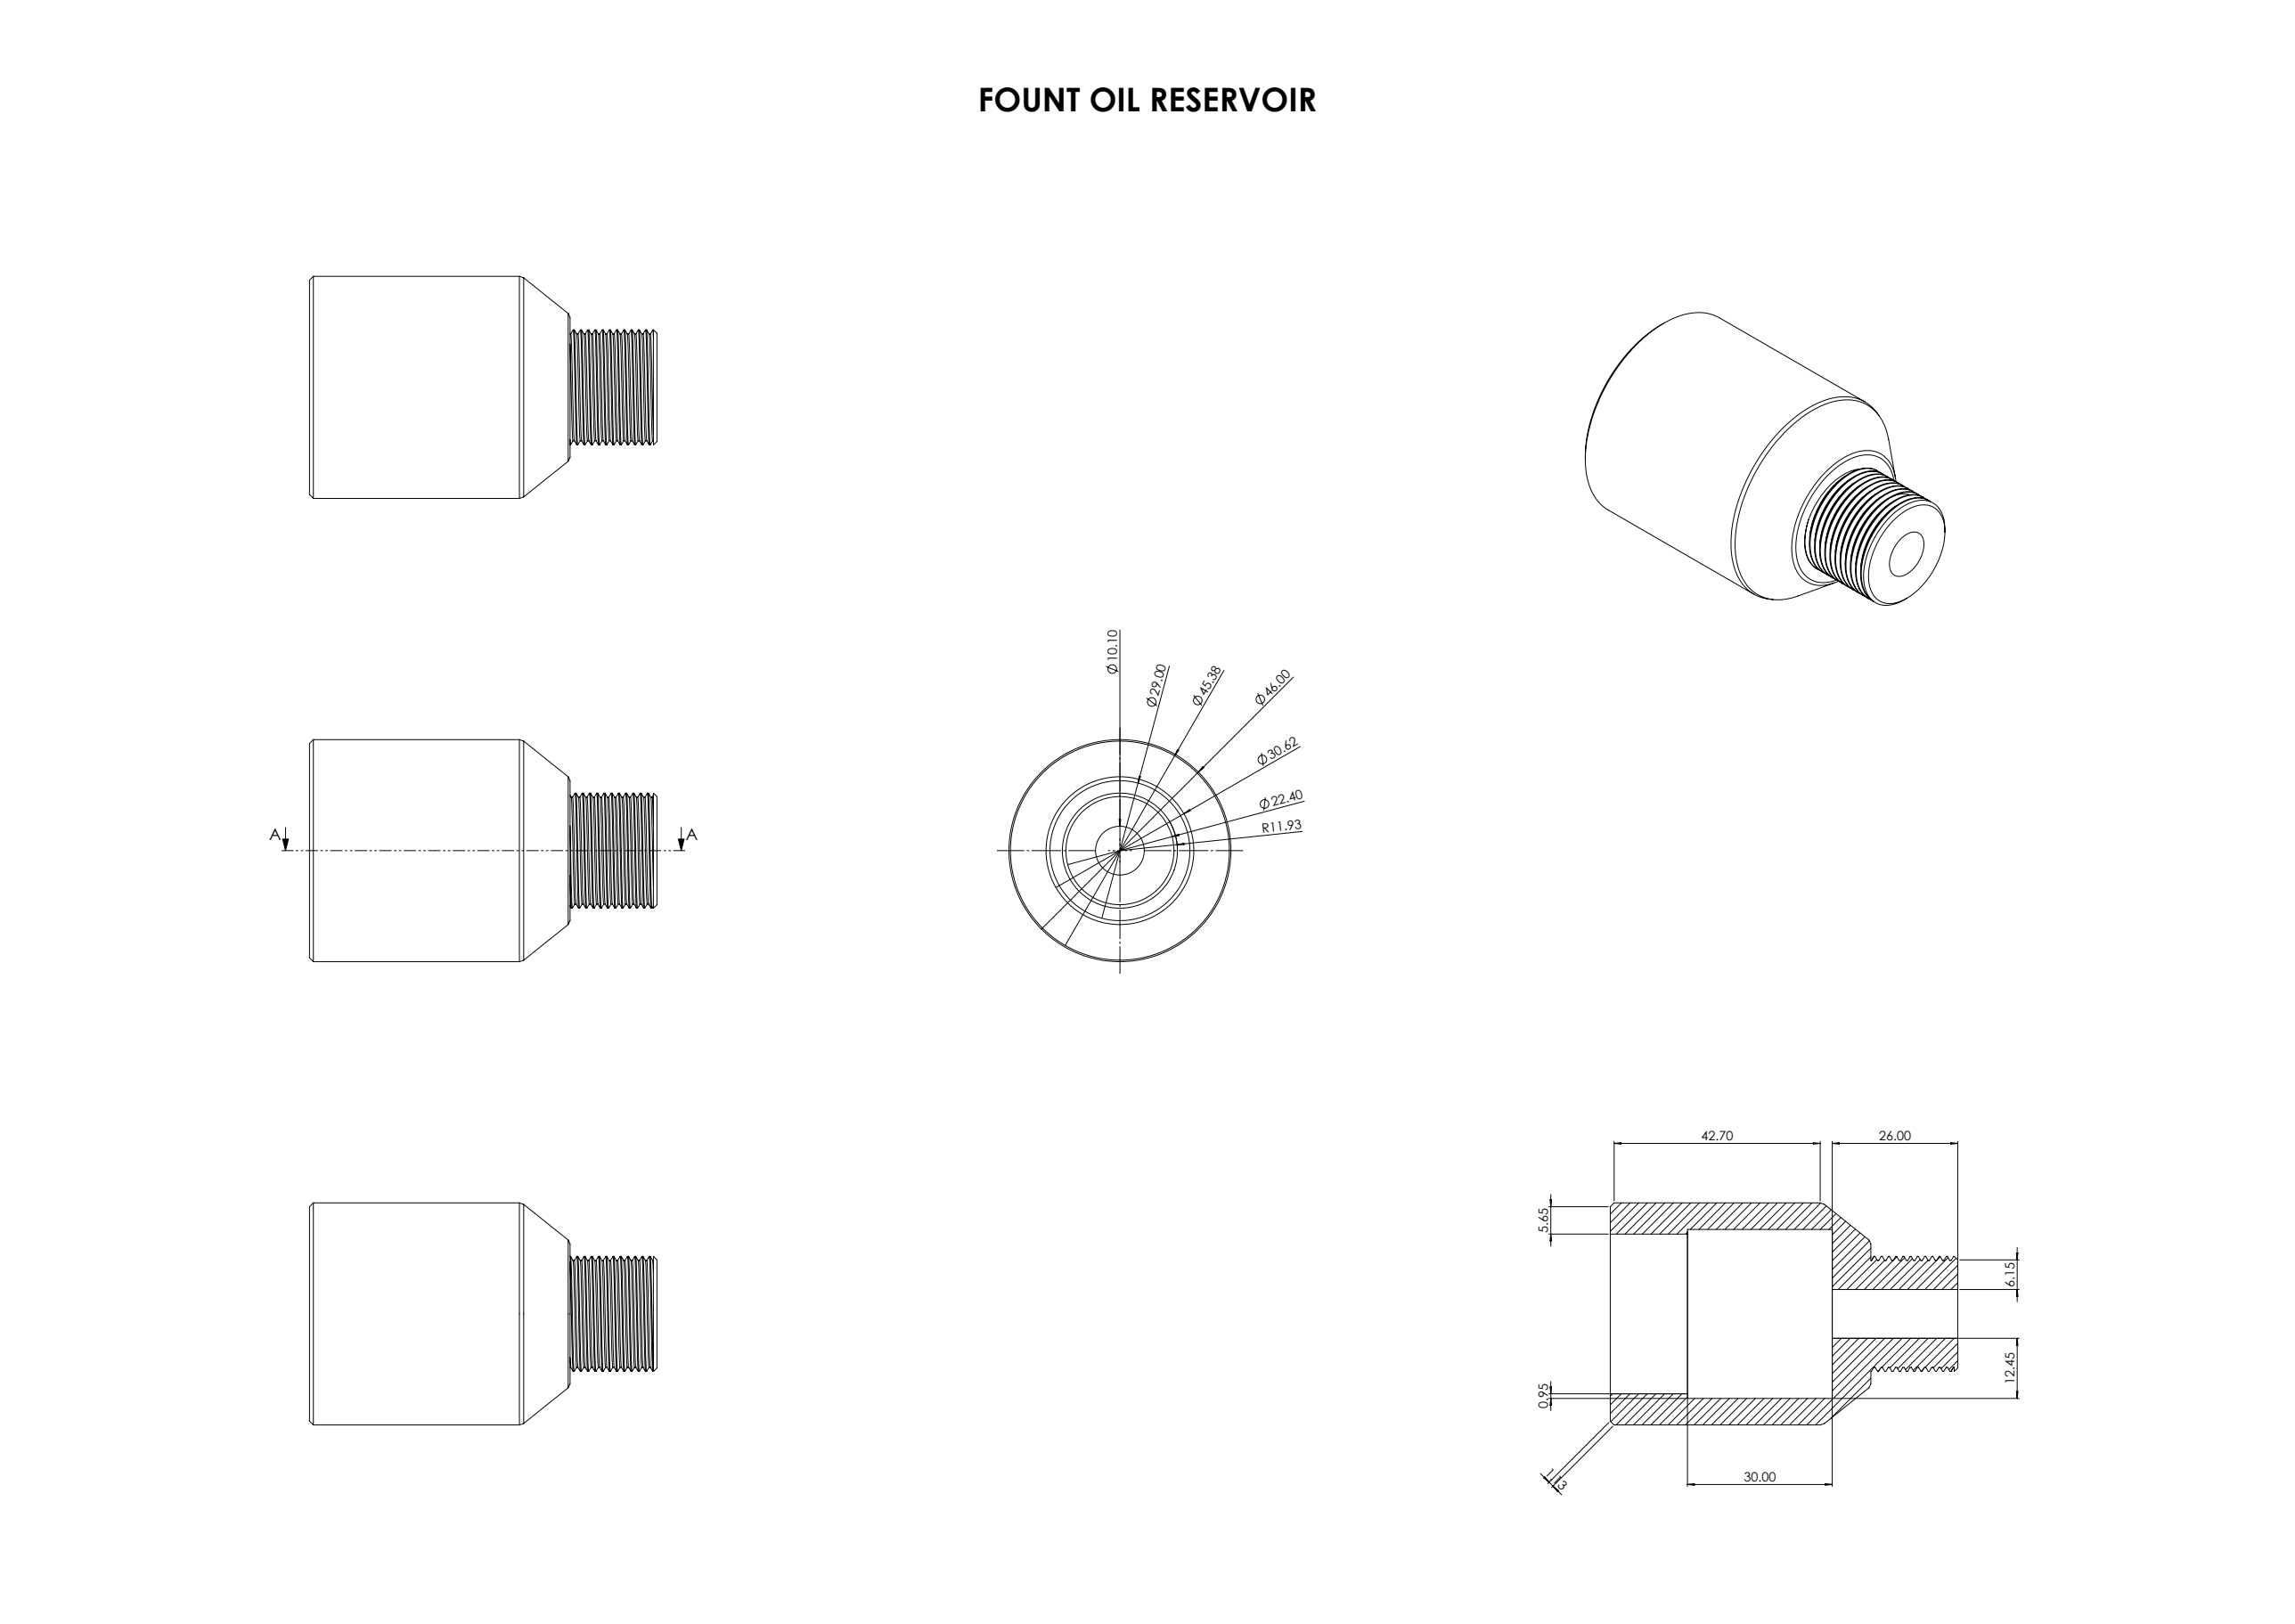
ISO-10303-21;
HEADER;
/* Generated by software containing ST-Developer
 * from STEP Tools, Inc. (www.steptools.com) 
 */

FILE_DESCRIPTION(
/* description */ (''),
/* implementation_level */ '2;1');

FILE_NAME(
/* name */ '16_Fount_Oil_Reservoir.step',
/* time_stamp */ '2026-10-26T03:55:20-07:00',
/* author */ (''),
/* organization */ (''),
/* preprocessor_version */ 'ST-DEVELOPER v20.2',
/* originating_system */ 'Autodesk Translation Framework v15.15.0.0',
/* authorisation */ '');

FILE_SCHEMA (('AUTOMOTIVE_DESIGN { 1 0 10303 214 3 1 1 }'));
ENDSEC;

DATA;
#10=MECHANICAL_DESIGN_GEOMETRIC_PRESENTATION_REPRESENTATION('',(#184),#45236);
#144=SHAPE_REPRESENTATION_RELATIONSHIP('SRR','None',#45323,#164);
#164=ADVANCED_BREP_SHAPE_REPRESENTATION('',(#204),#45225);
#184=STYLED_ITEM('',(#45498),#204);
#204=MANIFOLD_SOLID_BREP('Body1',#16526);
#575=B_SPLINE_CURVE_WITH_KNOTS('',3,(#33394,#33395,#33396,#33397,#33398,
#33399,#33400,#33401,#33402,#33403,#33404,#33405,#33406,#33407,#33408,#33409),
 .UNSPECIFIED.,.F.,.F.,(4,3,3,3,3,4),(-4.0929908801096,-3.9700734175722,
-3.47381424037567,-2.97755506317915,-2.48129588598262,-2.07752579179387),
 .UNSPECIFIED.);
#576=B_SPLINE_CURVE_WITH_KNOTS('',3,(#33412,#33413,#33414,#33415,#33416,
#33417,#33418,#33419,#33420,#33421),.UNSPECIFIED.,.F.,.F.,(4,3,3,4),(0.,
0.496259177196522,0.992518354393046,1.12612756527419),.UNSPECIFIED.);
#577=B_SPLINE_CURVE_WITH_KNOTS('',3,(#33426,#33427,#33428,#33429,#33430,
#33431,#33432,#33433,#33434,#33435,#33436,#33437,#33438,#33439,#33440,#33441,
#33442,#33443,#33444,#33445,#33446,#33447,#33448,#33449,#33450,#33451,#33452,
#33453,#33454,#33455,#33456,#33457,#33458,#33459,#33460,#33461,#33462,#33463,
#33464,#33465),.UNSPECIFIED.,.F.,.F.,(4,3,3,3,3,3,3,3,3,3,3,3,3,4),(-10.3761761872891,
-9.92518354393049,-9.42892436673396,-8.93266518953744,-8.43640601234091,
-7.94014683514439,-7.44388765794787,-6.94762848075134,-6.45136930355482,
-5.95511012635829,-5.45885094916177,-4.96259177196524,-4.46633259476872,
-4.0929908801096),.UNSPECIFIED.);
#578=B_SPLINE_CURVE_WITH_KNOTS('',3,(#33466,#33467,#33468,#33469,#33470,
#33471,#33472,#33473,#33474,#33475,#33476,#33477,#33478,#33479,#33480,#33481,
#33482,#33483,#33484,#33485,#33486,#33487,#33488,#33489,#33490,#33491,#33492,
#33493,#33494,#33495,#33496,#33497,#33498,#33499,#33500,#33501,#33502,#33503,
#33504,#33505),.UNSPECIFIED.,.F.,.F.,(4,3,3,3,3,3,3,3,3,3,3,3,3,4),(1.12612756527419,
1.48877753158957,1.9850367087861,2.48129588598262,2.97755506317914,3.47381424037567,
3.97007341757219,4.46633259476871,4.96259177196524,5.45885094916176,5.95511012635829,
6.45136930355481,6.94762848075133,7.40931287245371),.UNSPECIFIED.);
#579=B_SPLINE_CURVE_WITH_KNOTS('',3,(#33510,#33511,#33512,#33513,#33514,
#33515,#33516,#33517,#33518,#33519,#33520,#33521,#33522,#33523,#33524,#33525,
#33526,#33527,#33528,#33529,#33530,#33531,#33532,#33533,#33534,#33535,#33536,
#33537,#33538,#33539,#33540,#33541,#33542,#33543,#33544,#33545,#33546,#33547,
#33548,#33549,#33550,#33551,#33552),.UNSPECIFIED.,.F.,.F.,(4,3,3,3,3,3,
3,3,3,3,3,3,3,3,4),(-16.6593614944688,-16.3765528474853,-15.8802936702888,
-15.3840344930923,-14.8877753158957,-14.3915161386992,-13.8952569615027,
-13.3989977843062,-12.9027386071096,-12.4064794299131,-11.9102202527166,
-11.4139610755201,-10.9177018983235,-10.421442721127,-10.3761761872891),
 .UNSPECIFIED.);
#580=B_SPLINE_CURVE_WITH_KNOTS('',3,(#33553,#33554,#33555,#33556,#33557,
#33558,#33559,#33560,#33561,#33562,#33563,#33564,#33565,#33566,#33567,#33568,
#33569,#33570,#33571,#33572,#33573,#33574,#33575,#33576,#33577,#33578,#33579,
#33580,#33581,#33582,#33583,#33584,#33585,#33586,#33587,#33588,#33589,#33590,
#33591,#33592,#33593,#33594,#33595),.UNSPECIFIED.,.F.,.F.,(4,3,3,3,3,3,
3,3,3,3,3,3,3,3,4),(7.40931287245371,7.44388765794786,7.94014683514438,
8.43640601234091,8.93266518953743,9.42892436673395,9.92518354393048,10.421442721127,
10.9177018983235,11.41396107552,11.9102202527166,12.4064794299131,12.9027386071096,
13.3989977843061,13.6924981796334),.UNSPECIFIED.);
#581=B_SPLINE_CURVE_WITH_KNOTS('',3,(#33600,#33601,#33602,#33603,#33604,
#33605,#33606,#33607,#33608,#33609,#33610,#33611,#33612,#33613,#33614,#33615,
#33616,#33617,#33618,#33619,#33620,#33621,#33622,#33623,#33624,#33625,#33626,
#33627,#33628,#33629,#33630,#33631,#33632,#33633,#33634,#33635,#33636,#33637,
#33638,#33639,#33640,#33641,#33642),.UNSPECIFIED.,.F.,.F.,(4,3,3,3,3,3,
3,3,3,3,3,3,3,3,4),(-22.9425468016483,-22.8279221510401,-22.3316629738436,
-21.8354037966471,-21.3391446194506,-20.842885442254,-20.3466262650575,
-19.850367087861,-19.3541079106645,-18.8578487334679,-18.3615895562714,
-17.8653303790749,-17.3690712018784,-16.8728120246818,-16.6593614944688),
 .UNSPECIFIED.);
#582=B_SPLINE_CURVE_WITH_KNOTS('',3,(#33643,#33644,#33645,#33646,#33647,
#33648,#33649,#33650,#33651,#33652,#33653,#33654,#33655,#33656,#33657,#33658,
#33659,#33660,#33661,#33662,#33663,#33664,#33665,#33666,#33667,#33668,#33669,
#33670,#33671,#33672,#33673,#33674,#33675,#33676,#33677,#33678,#33679,#33680,
#33681,#33682,#33683,#33684,#33685),.UNSPECIFIED.,.F.,.F.,(4,3,3,3,3,3,
3,3,3,3,3,3,3,3,4),(13.6924981796334,13.8952569615027,14.3915161386992,
14.8877753158957,15.3840344930922,15.8802936702888,16.3765528474853,16.8728120246818,
17.3690712018783,17.8653303790749,18.3615895562714,18.8578487334679,19.3541079106644,
19.850367087861,19.9756834868129),.UNSPECIFIED.);
#583=B_SPLINE_CURVE_WITH_KNOTS('',3,(#33690,#33691,#33692,#33693,#33694,
#33695,#33696,#33697,#33698,#33699,#33700,#33701,#33702,#33703,#33704,#33705,
#33706,#33707,#33708,#33709,#33710,#33711,#33712,#33713,#33714,#33715,#33716,
#33717,#33718,#33719,#33720,#33721,#33722,#33723,#33724,#33725,#33726,#33727,
#33728,#33729),.UNSPECIFIED.,.F.,.F.,(4,3,3,3,3,3,3,3,3,3,3,3,3,4),(-29.2257321088278,
-28.7830322773984,-28.2867731002019,-27.7905139230054,-27.2942547458088,
-26.7979955686123,-26.3017363914158,-25.8054772142193,-25.3092180370227,
-24.8129588598262,-24.3166996826297,-23.8204405054332,-23.3241813282366,
-22.9425468016483),.UNSPECIFIED.);
#584=B_SPLINE_CURVE_WITH_KNOTS('',3,(#33730,#33731,#33732,#33733,#33734,
#33735,#33736,#33737,#33738,#33739,#33740,#33741,#33742,#33743,#33744,#33745,
#33746,#33747,#33748,#33749,#33750,#33751,#33752,#33753,#33754,#33755,#33756,
#33757,#33758,#33759,#33760,#33761,#33762,#33763,#33764,#33765,#33766,#33767,
#33768,#33769),.UNSPECIFIED.,.F.,.F.,(4,3,3,3,3,3,3,3,3,3,3,3,3,4),(19.9756834868129,
20.3466262650575,20.842885442254,21.3391446194505,21.8354037966471,22.3316629738436,
22.8279221510401,23.3241813282366,23.8204405054331,24.3166996826297,24.8129588598262,
25.3092180370227,25.8054772142192,26.2588687939926),.UNSPECIFIED.);
#585=B_SPLINE_CURVE_WITH_KNOTS('',3,(#33774,#33775,#33776,#33777,#33778,
#33779,#33780,#33781,#33782,#33783,#33784,#33785,#33786,#33787,#33788,#33789,
#33790,#33791,#33792,#33793,#33794,#33795,#33796,#33797,#33798,#33799,#33800,
#33801,#33802,#33803,#33804,#33805,#33806,#33807,#33808,#33809,#33810,#33811,
#33812,#33813,#33814,#33815,#33816),.UNSPECIFIED.,.F.,.F.,(4,3,3,3,3,3,
3,3,3,3,3,3,3,3,4),(-35.5089174160075,-35.2344015809532,-34.7381424037567,
-34.2418832265602,-33.7456240493637,-33.2493648721671,-32.7531056949706,
-32.2568465177741,-31.7605873405776,-31.264328163381,-30.7680689861845,
-30.271809808988,-29.7755506317915,-29.2792914545949,-29.2257321088278),
 .UNSPECIFIED.);
#586=B_SPLINE_CURVE_WITH_KNOTS('',3,(#33817,#33818,#33819,#33820,#33821,
#33822,#33823,#33824,#33825,#33826,#33827,#33828,#33829,#33830,#33831,#33832,
#33833,#33834,#33835,#33836,#33837,#33838,#33839,#33840,#33841,#33842,#33843,
#33844,#33845,#33846,#33847,#33848,#33849,#33850,#33851,#33852,#33853,#33854,
#33855,#33856,#33857,#33858,#33859),.UNSPECIFIED.,.F.,.F.,(4,3,3,3,3,3,
3,3,3,3,3,3,3,3,4),(26.2588687939926,26.3017363914158,26.7979955686123,
27.2942547458088,27.7905139230053,28.2867731002019,28.7830322773984,29.2792914545949,
29.7755506317914,30.271809808988,30.7680689861845,31.264328163381,31.7605873405775,
32.2568465177741,32.5420541011721),.UNSPECIFIED.);
#587=B_SPLINE_CURVE_WITH_KNOTS('',3,(#33864,#33865,#33866,#33867,#33868,
#33869,#33870,#33871,#33872,#33873,#33874,#33875,#33876,#33877,#33878,#33879,
#33880,#33881,#33882,#33883,#33884,#33885,#33886,#33887,#33888,#33889,#33890,
#33891,#33892,#33893,#33894,#33895,#33896,#33897,#33898,#33899,#33900,#33901,
#33902,#33903,#33904,#33905,#33906),.UNSPECIFIED.,.F.,.F.,(4,3,3,3,3,3,
3,3,3,3,3,3,3,3,4),(-41.792102723187,-41.685770884508,-41.1895117073115,
-40.693252530115,-40.1969933529185,-39.700734175722,-39.2044749985254,-38.7082158213289,
-38.2119566441324,-37.7156974669359,-37.2194382897393,-36.7231791125428,
-36.2269199353463,-35.7306607581498,-35.5089174160075),.UNSPECIFIED.);
#588=B_SPLINE_CURVE_WITH_KNOTS('',3,(#33907,#33908,#33909,#33910,#33911,
#33912,#33913,#33914,#33915,#33916,#33917,#33918,#33919,#33920,#33921,#33922,
#33923,#33924,#33925,#33926,#33927,#33928,#33929,#33930,#33931,#33932,#33933,
#33934,#33935,#33936,#33937,#33938,#33939,#33940,#33941,#33942,#33943,#33944,
#33945,#33946,#33947,#33948,#33949),.UNSPECIFIED.,.F.,.F.,(4,3,3,3,3,3,
3,3,3,3,3,3,3,3,4),(32.5420541011721,32.7531056949706,33.2493648721671,
33.7456240493636,34.2418832265602,34.7381424037567,35.2344015809532,35.7306607581497,
36.2269199353462,36.7231791125428,37.2194382897393,37.7156974669358,38.2119566441323,
38.7082158213289,38.8252394083516),.UNSPECIFIED.);
#589=B_SPLINE_CURVE_WITH_KNOTS('',3,(#33954,#33955,#33956,#33957,#33958,
#33959,#33960,#33961,#33962,#33963,#33964,#33965,#33966,#33967,#33968,#33969,
#33970,#33971,#33972,#33973,#33974,#33975,#33976,#33977,#33978,#33979,#33980,
#33981,#33982,#33983,#33984,#33985,#33986,#33987,#33988,#33989,#33990,#33991,
#33992,#33993),.UNSPECIFIED.,.F.,.F.,(4,3,3,3,3,3,3,3,3,3,3,3,3,4),(-48.0752880303667,
-47.6408810108663,-47.1446218336698,-46.6483626564733,-46.1521034792768,
-45.6558443020802,-45.1595851248837,-44.6633259476872,-44.1670667704907,
-43.6708075932941,-43.1745484160976,-42.6782892389011,-42.1820300617046,
-41.792102723187),.UNSPECIFIED.);
#590=B_SPLINE_CURVE_WITH_KNOTS('',3,(#33994,#33995,#33996,#33997,#33998,
#33999,#34000,#34001,#34002,#34003,#34004,#34005,#34006,#34007,#34008,#34009,
#34010,#34011,#34012,#34013,#34014,#34015,#34016,#34017,#34018,#34019,#34020,
#34021,#34022,#34023,#34024,#34025,#34026,#34027,#34028,#34029,#34030,#34031,
#34032,#34033),.UNSPECIFIED.,.F.,.F.,(4,3,3,3,3,3,3,3,3,3,3,3,3,4),(38.8252394083516,
39.2044749985254,39.7007341757219,40.1969933529184,40.693252530115,41.1895117073115,
41.685770884508,42.1820300617045,42.678289238901,43.1745484160976,43.6708075932941,
44.1670667704906,44.6633259476871,45.1084247155313),.UNSPECIFIED.);
#591=B_SPLINE_CURVE_WITH_KNOTS('',3,(#34038,#34039,#34040,#34041,#34042,
#34043,#34044,#34045,#34046,#34047,#34048,#34049,#34050,#34051,#34052,#34053,
#34054,#34055,#34056,#34057,#34058,#34059,#34060,#34061,#34062,#34063,#34064,
#34065,#34066,#34067,#34068,#34069,#34070,#34071,#34072,#34073,#34074,#34075,
#34076,#34077,#34078,#34079,#34080),.UNSPECIFIED.,.F.,.F.,(4,3,3,3,3,3,
3,3,3,3,3,3,3,3,4),(-54.3584733375463,-54.0922503144212,-53.5959911372246,
-53.0997319600281,-52.6034727828316,-52.1072136056351,-51.6109544284385,
-51.114695251242,-50.6184360740455,-50.122176896849,-49.6259177196524,-49.1296585424559,
-48.6333993652594,-48.1371401880629,-48.0752880303667),.UNSPECIFIED.);
#592=B_SPLINE_CURVE_WITH_KNOTS('',3,(#34081,#34082,#34083,#34084,#34085,
#34086,#34087,#34088,#34089,#34090,#34091,#34092,#34093,#34094,#34095,#34096,
#34097,#34098,#34099,#34100,#34101,#34102,#34103,#34104,#34105,#34106,#34107,
#34108,#34109,#34110,#34111,#34112,#34113,#34114,#34115,#34116,#34117,#34118,
#34119,#34120,#34121,#34122,#34123),.UNSPECIFIED.,.F.,.F.,(4,3,3,3,3,3,
3,3,3,3,3,3,3,3,4),(45.1084247155313,45.1595851248837,45.6558443020802,
46.1521034792767,46.6483626564732,47.1446218336698,47.6408810108663,48.1371401880628,
48.6333993652593,49.1296585424559,49.6259177196524,50.1221768968489,50.6184360740454,
51.114695251242,51.3916100227108),.UNSPECIFIED.);
#593=B_SPLINE_CURVE_WITH_KNOTS('',3,(#34128,#34129,#34130,#34131,#34132,
#34133,#34134,#34135,#34136,#34137,#34138,#34139,#34140,#34141,#34142,#34143,
#34144,#34145,#34146,#34147,#34148,#34149,#34150,#34151,#34152,#34153,#34154,
#34155,#34156,#34157,#34158,#34159,#34160,#34161,#34162,#34163,#34164,#34165,
#34166,#34167,#34168,#34169,#34170),.UNSPECIFIED.,.F.,.F.,(4,3,3,3,3,3,
3,3,3,3,3,3,3,3,4),(-60.6416586447259,-60.543619617976,-60.0473604407794,
-59.5511012635829,-59.0548420863864,-58.5585829091899,-58.0623237319934,
-57.5660645547968,-57.0698053776003,-56.5735462004038,-56.0772870232073,
-55.5810278460107,-55.0847686688142,-54.5885094916177,-54.3584733375463),
 .UNSPECIFIED.);
#594=B_SPLINE_CURVE_WITH_KNOTS('',3,(#34171,#34172,#34173,#34174,#34175,
#34176,#34177,#34178,#34179,#34180,#34181,#34182,#34183,#34184,#34185,#34186,
#34187,#34188,#34189,#34190,#34191,#34192,#34193,#34194,#34195,#34196,#34197,
#34198,#34199,#34200,#34201,#34202,#34203,#34204,#34205,#34206,#34207,#34208,
#34209,#34210,#34211,#34212,#34213),.UNSPECIFIED.,.F.,.F.,(4,3,3,3,3,3,
3,3,3,3,3,3,3,3,4),(51.3916100227108,51.6109544284385,52.107213605635,52.6034727828315,
53.0997319600281,53.5959911372246,54.0922503144211,54.5885094916176,55.0847686688141,
55.5810278460107,56.0772870232072,56.5735462004037,57.0698053776003,57.5660645547968,
57.6747953298905),.UNSPECIFIED.);
#595=B_SPLINE_CURVE_WITH_KNOTS('',3,(#34218,#34219,#34220,#34221,#34222,
#34223,#34224,#34225,#34226,#34227,#34228,#34229,#34230,#34231,#34232,#34233,
#34234,#34235,#34236,#34237,#34238,#34239,#34240,#34241,#34242,#34243,#34244,
#34245,#34246,#34247,#34248,#34249,#34250,#34251,#34252,#34253,#34254,#34255,
#34256,#34257),.UNSPECIFIED.,.F.,.F.,(4,3,3,3,3,3,3,3,3,3,3,3,3,4),(-66.9248439519054,
-66.4987297443343,-66.0024705671378,-65.5062113899412,-65.0099522127447,
-64.5136930355482,-64.0174338583517,-63.5211746811551,-63.0249155039586,
-62.5286563267621,-62.0323971495656,-61.536137972369,-61.0398787951725,
-60.6416586447259),.UNSPECIFIED.);
#596=B_SPLINE_CURVE_WITH_KNOTS('',3,(#34258,#34259,#34260,#34261,#34262,
#34263,#34264,#34265,#34266,#34267,#34268,#34269,#34270,#34271,#34272,#34273,
#34274,#34275,#34276,#34277,#34278,#34279,#34280,#34281,#34282,#34283,#34284,
#34285,#34286,#34287,#34288,#34289,#34290,#34291,#34292,#34293,#34294,#34295,
#34296,#34297),.UNSPECIFIED.,.F.,.F.,(4,3,3,3,3,3,3,3,3,3,3,3,3,4),(57.6747953298905,
58.0623237319933,58.5585829091898,59.0548420863863,59.5511012635829,60.0473604407794,
60.5436196179759,61.0398787951725,61.536137972369,62.0323971495655,62.528656326762,
63.0249155039585,63.5211746811551,63.95798063707),.UNSPECIFIED.);
#597=B_SPLINE_CURVE_WITH_KNOTS('',3,(#34302,#34303,#34304,#34305,#34306,
#34307,#34308,#34309,#34310,#34311,#34312,#34313,#34314,#34315,#34316,#34317,
#34318,#34319,#34320,#34321,#34322,#34323,#34324,#34325,#34326,#34327,#34328,
#34329,#34330,#34331,#34332,#34333,#34334,#34335,#34336,#34337,#34338,#34339,
#34340,#34341,#34342,#34343,#34344),.UNSPECIFIED.,.F.,.F.,(4,3,3,3,3,3,
3,3,3,3,3,3,3,3,4),(-73.2080292590851,-72.9500990478891,-72.4538398706926,
-71.957580693496,-71.4613215162995,-70.965062339103,-70.4688031619065,-69.97254398471,
-69.4762848075134,-68.9800256303169,-68.4837664531204,-67.9875072759238,
-67.4912480987273,-66.9949889215308,-66.9248439519054),.UNSPECIFIED.);
#598=B_SPLINE_CURVE_WITH_KNOTS('',3,(#34345,#34346,#34347,#34348,#34349,
#34350,#34351,#34352,#34353,#34354,#34355,#34356,#34357,#34358,#34359,#34360,
#34361,#34362,#34363,#34364,#34365,#34366,#34367,#34368,#34369,#34370,#34371,
#34372,#34373,#34374,#34375,#34376,#34377,#34378,#34379,#34380,#34381,#34382,
#34383,#34384,#34385,#34386,#34387),.UNSPECIFIED.,.F.,.F.,(4,3,3,3,3,3,
3,3,3,3,3,3,3,3,4),(63.95798063707,64.0174338583516,64.5136930355481,65.0099522127446,
65.5062113899412,66.0024705671377,66.4987297443342,66.9949889215307,67.4912480987273,
67.9875072759238,68.4837664531203,68.9800256303168,69.4762848075134,69.9725439847099,
70.2411659442497),.UNSPECIFIED.);
#599=B_SPLINE_CURVE_WITH_KNOTS('',3,(#34393,#34394,#34395,#34396,#34397,
#34398,#34399,#34400,#34401,#34402,#34403,#34404,#34405,#34406,#34407),
 .UNSPECIFIED.,.F.,.F.,(4,1,1,1,1,1,1,1,1,1,1,1,4),(78.5398163397448,78.6099613093701,
79.1062204865667,79.6024796637632,80.0987388409597,80.5949980181562,81.0912571953528,
81.5875163725493,82.0837755497458,82.5800347269423,83.0762939041389,83.5725530813354,
83.9763231755241),.UNSPECIFIED.);
#600=B_SPLINE_CURVE_WITH_KNOTS('',3,(#34410,#34411,#34412,#34413,#34414,
#34415,#34416,#34417,#34418,#34419,#34420,#34421),.UNSPECIFIED.,.F.,.F.,
(4,1,1,1,1,1,1,1,1,4),(78.5398163397448,78.7674535574015,79.263712734598,
79.7599719117945,80.2562310889911,80.7524902661876,81.2487494433841,81.7450086205806,
82.2412677977772,82.7375269749737),.UNSPECIFIED.);
#601=B_SPLINE_CURVE_WITH_KNOTS('',3,(#34426,#34427,#34428,#34429,#34430,
#34431,#34432,#34433,#34434,#34435,#34436,#34437,#34438,#34439,#34440,#34441),
 .UNSPECIFIED.,.F.,.F.,(4,1,1,1,1,1,1,1,1,1,1,1,1,4),(72.2566310325653,
72.6548511830118,73.1511103602084,73.6473695374049,74.1436287146014,74.6398878917979,
75.1361470689945,75.632406246191,76.1286654233875,76.624924600584,77.1211837777806,
77.6174429549771,78.1137021321736,78.5398163397448),.UNSPECIFIED.);
#602=B_SPLINE_CURVE_WITH_KNOTS('',3,(#34442,#34443,#34444,#34445,#34446,
#34447,#34448,#34449,#34450,#34451,#34452,#34453,#34454,#34455,#34456,#34457,
#34458),.UNSPECIFIED.,.F.,.F.,(4,1,1,1,1,1,1,1,1,1,1,1,1,1,4),(72.2566310325653,
72.3160842538467,72.8123434310432,73.3086026082397,73.8048617854362,74.3011209626328,
74.7973801398293,75.2936393170258,75.7898984942223,76.2861576714189,76.7824168486154,
77.2786760258119,77.7749352030084,78.271194380205,78.5398163397448),
 .UNSPECIFIED.);
#603=B_SPLINE_CURVE_WITH_KNOTS('',3,(#34463,#34464,#34465,#34466,#34467,
#34468,#34469,#34470,#34471,#34472,#34473,#34474,#34475,#34476,#34477,#34478,
#34479),.UNSPECIFIED.,.F.,.F.,(4,1,1,1,1,1,1,1,1,1,1,1,1,1,4),(65.9734457253856,
66.203481879457,66.6997410566536,67.1960002338501,67.6922594110466,68.1885185882431,
68.6847777654396,69.1810369426362,69.6772961198327,70.1735552970292,70.6698144742257,
71.1660736514223,71.6623328286188,72.1585920058153,72.2566310325653),
 .UNSPECIFIED.);
#604=B_SPLINE_CURVE_WITH_KNOTS('',3,(#34480,#34481,#34482,#34483,#34484,
#34485,#34486,#34487,#34488,#34489,#34490,#34491,#34492,#34493,#34494,#34495),
 .UNSPECIFIED.,.F.,.F.,(4,1,1,1,1,1,1,1,1,1,1,1,1,4),(65.9734457253856,
66.3609741274884,66.8572333046849,67.3534924818814,67.849751659078,68.3460108362745,
68.842270013471,69.3385291906675,69.8347883678641,70.3310475450606,70.8273067222571,
71.3235658994536,71.8198250766501,72.2566310325653),.UNSPECIFIED.);
#605=B_SPLINE_CURVE_WITH_KNOTS('',3,(#34500,#34501,#34502,#34503,#34504,
#34505,#34506,#34507,#34508,#34509,#34510,#34511,#34512,#34513,#34514,#34515,
#34516),.UNSPECIFIED.,.F.,.F.,(4,1,1,1,1,1,1,1,1,1,1,1,1,1,4),(59.6902604182061,
59.7521125759022,60.2483717530987,60.7446309302953,61.2408901074918,61.7371492846883,
62.2334084618848,62.7296676390814,63.2259268162779,63.7221859934744,64.2184451706709,
64.7147043478674,65.210963525064,65.7072227022605,65.9734457253856),
 .UNSPECIFIED.);
#606=B_SPLINE_CURVE_WITH_KNOTS('',3,(#34517,#34518,#34519,#34520,#34521,
#34522,#34523,#34524,#34525,#34526,#34527,#34528,#34529,#34530,#34531,#34532,
#34533),.UNSPECIFIED.,.F.,.F.,(4,1,1,1,1,1,1,1,1,1,1,1,1,1,4),(59.6902604182061,
59.9096048239336,60.4058640011301,60.9021231783266,61.3983823555232,61.8946415327197,
62.3909007099162,62.8871598871127,63.3834190643093,63.8796782415058,64.3759374187023,
64.8721965958988,65.3684557730953,65.8647149502919,65.9734457253856),
 .UNSPECIFIED.);
#607=B_SPLINE_CURVE_WITH_KNOTS('',3,(#34538,#34539,#34540,#34541,#34542,
#34543,#34544,#34545,#34546,#34547,#34548,#34549,#34550,#34551,#34552,#34553),
 .UNSPECIFIED.,.F.,.F.,(4,1,1,1,1,1,1,1,1,1,1,1,1,4),(53.4070751110264,
53.7970024495439,54.2932616267404,54.789520803937,55.2857799811335,55.78203915833,
56.2782983355265,56.7745575127231,57.2708166899196,57.7670758671161,58.2633350443126,
58.7595942215092,59.2558533987057,59.6902604182061),.UNSPECIFIED.);
#608=B_SPLINE_CURVE_WITH_KNOTS('',3,(#34554,#34555,#34556,#34557,#34558,
#34559,#34560,#34561,#34562,#34563,#34564,#34565,#34566,#34567,#34568,#34569,
#34570),.UNSPECIFIED.,.F.,.F.,(4,1,1,1,1,1,1,1,1,1,1,1,1,1,4),(53.4070751110264,
53.4582355203788,53.9544946975753,54.4507538747718,54.9470130519683,55.4432722291649,
55.9395314063614,56.4357905835579,56.9320497607544,57.428308937951,57.9245681151475,
58.420827292344,58.9170864695405,59.4133456467371,59.6902604182061),
 .UNSPECIFIED.);
#609=B_SPLINE_CURVE_WITH_KNOTS('',3,(#34575,#34576,#34577,#34578,#34579,
#34580,#34581,#34582,#34583,#34584,#34585,#34586,#34587,#34588,#34589,#34590,
#34591),.UNSPECIFIED.,.F.,.F.,(4,1,1,1,1,1,1,1,1,1,1,1,1,1,4),(47.1238898038469,
47.3456331459891,47.8418923231856,48.3381515003821,48.8344106775787,49.3306698547752,
49.8269290319717,50.3231882091682,50.8194473863648,51.3157065635613,51.8119657407578,
52.3082249179543,52.8044840951509,53.3007432723474,53.4070751110264),
 .UNSPECIFIED.);
#610=B_SPLINE_CURVE_WITH_KNOTS('',3,(#34592,#34593,#34594,#34595,#34596,
#34597,#34598,#34599,#34600,#34601,#34602,#34603,#34604,#34605,#34606,#34607),
 .UNSPECIFIED.,.F.,.F.,(4,1,1,1,1,1,1,1,1,1,1,1,1,4),(47.1238898038469,
47.5031253940205,47.999384571217,48.4956437484135,48.9919029256101,49.4881621028066,
49.9844212800031,50.4806804571996,50.9769396343962,51.4731988115927,51.9694579887892,
52.4657171659857,52.9619763431823,53.4070751110264),.UNSPECIFIED.);
#611=B_SPLINE_CURVE_WITH_KNOTS('',3,(#34612,#34613,#34614,#34615,#34616,
#34617,#34618,#34619,#34620,#34621,#34622,#34623,#34624,#34625,#34626,#34627,
#34628),.UNSPECIFIED.,.F.,.F.,(4,1,1,1,1,1,1,1,1,1,1,1,1,1,4),(40.8407044966672,
40.8942638424343,41.3905230196308,41.8867821968273,42.3830413740238,42.8793005512204,
43.3755597284169,43.8718189056134,44.36807808281,44.8643372600065,45.360596437203,
45.8568556143995,46.353114791596,46.8493739687926,47.1238898038469),
 .UNSPECIFIED.);
#612=B_SPLINE_CURVE_WITH_KNOTS('',3,(#34629,#34630,#34631,#34632,#34633,
#34634,#34635,#34636,#34637,#34638,#34639,#34640,#34641,#34642,#34643,#34644,
#34645),.UNSPECIFIED.,.F.,.F.,(4,1,1,1,1,1,1,1,1,1,1,1,1,1,4),(40.8407044966672,
41.0517560904657,41.5480152676622,42.0442744448587,42.5405336220552,43.0367927992518,
43.5330519764483,44.0293111536448,44.5255703308413,45.0218295080379,45.5180886852344,
46.0143478624309,46.5106070396274,47.006866216824,47.1238898038469),
 .UNSPECIFIED.);
#613=B_SPLINE_CURVE_WITH_KNOTS('',3,(#34650,#34651,#34652,#34653,#34654,
#34655,#34656,#34657,#34658,#34659,#34660,#34661,#34662,#34663,#34664,#34665),
 .UNSPECIFIED.,.F.,.F.,(4,1,1,1,1,1,1,1,1,1,1,1,1,4),(34.5575191894877,
34.939153716076,35.4354128932725,35.931672070469,36.4279312476656,36.9241904248621,
37.4204496020586,37.9167087792551,38.4129679564517,38.9092271336482,39.4054863108447,
39.9017454880412,40.3980046652377,40.8407044966672),.UNSPECIFIED.);
#614=B_SPLINE_CURVE_WITH_KNOTS('',3,(#34666,#34667,#34668,#34669,#34670,
#34671,#34672,#34673,#34674,#34675,#34676,#34677,#34678,#34679,#34680,#34681,
#34682),.UNSPECIFIED.,.F.,.F.,(4,1,1,1,1,1,1,1,1,1,1,1,1,1,4),(34.5575191894877,
34.6003867869109,35.0966459641074,35.5929051413039,36.0891643185004,36.585423495697,
37.0816826728935,37.57794185009,38.0742010272865,38.5704602044831,39.0667193816796,
39.5629785588761,40.0592377360726,40.5554969132692,40.8407044966672),
 .UNSPECIFIED.);
#615=B_SPLINE_CURVE_WITH_KNOTS('',3,(#34687,#34688,#34689,#34690,#34691,
#34692,#34693,#34694,#34695,#34696,#34697,#34698,#34699,#34700,#34701,#34702,
#34703),.UNSPECIFIED.,.F.,.F.,(4,1,1,1,1,1,1,1,1,1,1,1,1,1,4),(28.2743338823082,
28.4877844125212,28.9840435897177,29.4803027669142,29.9765619441107,30.4728211213073,
30.9690802985038,31.4653394757003,31.9615986528968,32.4578578300934,32.9541170072899,
33.4503761844864,33.9466353616829,34.4428945388795,34.5575191894877),
 .UNSPECIFIED.);
#616=B_SPLINE_CURVE_WITH_KNOTS('',3,(#34704,#34705,#34706,#34707,#34708,
#34709,#34710,#34711,#34712,#34713,#34714,#34715,#34716,#34717,#34718,#34719),
 .UNSPECIFIED.,.F.,.F.,(4,1,1,1,1,1,1,1,1,1,1,1,1,4),(28.2743338823082,
28.6452766605526,29.1415358377491,29.6377950149456,30.1340541921422,30.6303133693387,
31.1265725465352,31.6228317237317,32.1190909009282,32.6153500781248,33.1116092553213,
33.6078684325178,34.1041276097143,34.5575191894877),.UNSPECIFIED.);
#617=B_SPLINE_CURVE_WITH_KNOTS('',3,(#34724,#34725,#34726,#34727,#34728,
#34729,#34730,#34731,#34732,#34733,#34734,#34735,#34736,#34737,#34738,#34739,
#34740),.UNSPECIFIED.,.F.,.F.,(4,1,1,1,1,1,1,1,1,1,1,1,1,1,4),(21.9911485751285,
22.0364151089663,22.5326742861629,23.0289334633594,23.5251926405559,24.0214518177524,
24.517710994949,25.0139701721455,25.510229349342,26.0064885265385,26.5027477037351,
26.9990068809316,27.4952660581281,27.9915252353246,28.2743338823082),
 .UNSPECIFIED.);
#618=B_SPLINE_CURVE_WITH_KNOTS('',3,(#34741,#34742,#34743,#34744,#34745,
#34746,#34747,#34748,#34749,#34750,#34751,#34752,#34753,#34754,#34755,#34756,
#34757),.UNSPECIFIED.,.F.,.F.,(4,1,1,1,1,1,1,1,1,1,1,1,1,1,4),(21.9911485751285,
22.1939073569978,22.6901665341943,23.1864257113908,23.6826848885873,24.1789440657839,
24.6752032429804,25.1714624201769,25.6677215973734,26.16398077457,26.6602399517665,
27.156499128963,27.6527583061595,28.1490174833561,28.2743338823082),
 .UNSPECIFIED.);
#619=B_SPLINE_CURVE_WITH_KNOTS('',3,(#34762,#34763,#34764,#34765,#34766,
#34767,#34768,#34769,#34770,#34771,#34772,#34773,#34774,#34775,#34776,#34777),
 .UNSPECIFIED.,.F.,.F.,(4,1,1,1,1,1,1,1,1,1,1,1,1,4),(15.707963267949,16.0813049826081,
16.5775641598046,17.0738233370011,17.5700825141976,18.0663416913942,18.5626008685907,
19.0588600457872,19.5551192229837,20.0513784001803,20.5476375773768,21.0438967545733,
21.5401559317698,21.9911485751285),.UNSPECIFIED.);
#620=B_SPLINE_CURVE_WITH_KNOTS('',3,(#34778,#34779,#34780,#34781,#34782,
#34783,#34784,#34785,#34786,#34787,#34788,#34789,#34790,#34791,#34792,#34793,
#34794),.UNSPECIFIED.,.F.,.F.,(4,1,1,1,1,1,1,1,1,1,1,1,1,1,4),(15.707963267949,
15.742538053443,16.2387972306395,16.735056407836,17.2313155850325,17.7275747622291,
18.2238339394256,18.7200931166221,19.2163522938186,19.7126114710152,20.2088706482117,
20.7051298254082,21.2013890026047,21.6976481798012,21.9911485751285),
 .UNSPECIFIED.);
#621=B_SPLINE_CURVE_WITH_KNOTS('',3,(#34811,#34812,#34813,#34814,#34815,
#34816,#34817,#34818,#34819,#34820,#34821,#34822,#34823,#34824,#34825,#34826,
#34827,#34828,#34829,#34830,#34831,#34832,#34833,#34834,#34835,#34836,#34837,
#34838,#34839,#34840,#34841,#34842,#34843,#34844,#34845,#34846,#34847,#34848,
#34849,#34850,#34851,#34852,#34853,#34854,#34855,#34856,#34857,#34858,#34859,
#34860,#34861,#34862,#34863,#34864,#34865,#34866,#34867,#34868,#34869,#34870,
#34871,#34872,#34873,#34874,#34875,#34876,#34877,#34878,#34879,#34880,#34881,
#34882,#34883,#34884,#34885,#34886,#34887,#34888,#34889,#34890,#34891,#34892,
#34893,#34894,#34895,#34896,#34897,#34898,#34899,#34900,#34901,#34902,#34903,
#34904,#34905,#34906,#34907,#34908,#34909,#34910,#34911,#34912,#34913,#34914,
#34915,#34916,#34917,#34918,#34919,#34920,#34921,#34922,#34923,#34924,#34925,
#34926,#34927,#34928,#34929,#34930,#34931,#34932,#34933,#34934,#34935,#34936,
#34937,#34938,#34939,#34940),.UNSPECIFIED.,.F.,.F.,(4,3,3,3,3,3,3,3,3,3,
3,3,3,3,3,3,3,3,3,3,3,3,3,3,3,3,3,3,3,3,3,3,3,3,3,3,3,3,3,3,3,3,3,4),(-2.39439908413783,
-2.30957055714608,-2.28423857194394,-2.1992123713416,-2.13667984916741,
-2.10464861416482,-2.08645022218986,-2.07576631254953,-1.99136800162839,
-1.90707270778559,-1.82339088190019,-1.79228120991215,-1.77736472887211,
-1.7676964721655,-1.69895219394804,-1.61556580382843,-1.5316846344345,-1.44789196762844,
-1.36656757104543,-1.33607092232681,-1.32613672030475,-1.31756701322122,
-1.23465419226132,-1.15190857282007,-1.12259438129642,-1.03956979703191,
-0.956697216050081,-0.906629990836835,-0.883172486284775,-0.870094147064423,
-0.788031684106132,-0.705898296538195,-0.624514288049676,-0.556159414344109,
-0.486639487551095,-0.456224519579152,-0.437728905707078,-0.429197413628179,
-0.348523537028714,-0.267263381794694,-0.186163914396806,-0.105687092063476,
-0.0266190971408737,0.),.UNSPECIFIED.);
#622=B_SPLINE_CURVE_WITH_KNOTS('',3,(#34943,#34944,#34945,#34946,#34947,
#34948,#34949,#34950,#34951,#34952,#34953,#34954,#34955,#34956,#34957,#34958,
#34959,#34960,#34961,#34962,#34963,#34964,#34965,#34966,#34967,#34968,#34969,
#34970,#34971,#34972,#34973,#34974,#34975,#34976,#34977,#34978,#34979,#34980,
#34981,#34982,#34983,#34984,#34985,#34986,#34987,#34988,#34989,#34990,#34991,
#34992,#34993,#34994,#34995,#34996,#34997,#34998,#34999,#35000,#35001,#35002,
#35003,#35004,#35005,#35006,#35007,#35008,#35009,#35010,#35011,#35012,#35013,
#35014,#35015,#35016,#35017,#35018,#35019,#35020,#35021,#35022,#35023,#35024,
#35025,#35026,#35027,#35028,#35029,#35030,#35031,#35032,#35033,#35034,#35035,
#35036,#35037,#35038,#35039,#35040,#35041,#35042,#35043,#35044,#35045,#35046,
#35047,#35048,#35049,#35050,#35051,#35052,#35053,#35054,#35055,#35056,#35057,
#35058,#35059,#35060,#35061,#35062,#35063,#35064,#35065,#35066,#35067,#35068,
#35069,#35070,#35071,#35072),.UNSPECIFIED.,.F.,.F.,(4,3,3,3,3,3,3,3,3,3,
3,3,3,3,3,3,3,3,3,3,3,3,3,3,3,3,3,3,3,3,3,3,3,3,3,3,3,3,3,3,3,3,3,4),(-2.39814946016208,
-2.31696204037272,-2.29529569174575,-2.21456972428986,-2.15490479428083,
-2.12648768752725,-2.10829922528945,-2.09678298213356,-2.01553459190536,
-1.93371848537121,-1.85215105787095,-1.82342586445762,-1.81332878484419,
-1.80373550389277,-1.73725028421764,-1.65586989418317,-1.57363756065892,
-1.49104149188928,-1.41031007232168,-1.38003578998382,-1.37054045619564,
-1.36256005099984,-1.27951391668103,-1.19605898221033,-1.16811581361885,
-1.08502370473436,-1.00162059695019,-0.950031361007238,-0.926067853715056,
-0.912515238783363,-0.828732204328819,-0.744476329949599,-0.660367719531965,
-0.588906709406546,-0.515293370730728,-0.483087535060058,-0.463174686736147,
-0.454053033267499,-0.370331877320448,-0.285650817662844,-0.200462204104426,
-0.115556056832656,-0.0317686426882691,0.),.UNSPECIFIED.);
#623=B_SPLINE_CURVE_WITH_KNOTS('',3,(#35085,#35086,#35087,#35088,#35089,
#35090,#35091,#35092,#35093,#35094,#35095,#35096,#35097,#35098,#35099,#35100,
#35101,#35102,#35103,#35104,#35105,#35106,#35107,#35108,#35109,#35110,#35111,
#35112,#35113,#35114,#35115,#35116,#35117,#35118,#35119,#35120,#35121,#35122,
#35123,#35124,#35125,#35126,#35127,#35128,#35129,#35130,#35131,#35132,#35133,
#35134,#35135,#35136,#35137,#35138,#35139,#35140,#35141,#35142,#35143,#35144,
#35145,#35146,#35147,#35148,#35149,#35150,#35151,#35152,#35153,#35154,#35155,
#35156,#35157,#35158,#35159,#35160,#35161,#35162,#35163,#35164,#35165,#35166,
#35167,#35168,#35169,#35170,#35171,#35172,#35173,#35174,#35175,#35176,#35177,
#35178,#35179,#35180,#35181,#35182,#35183,#35184,#35185,#35186,#35187,#35188,
#35189,#35190,#35191,#35192,#35193,#35194,#35195,#35196,#35197,#35198,#35199,
#35200,#35201,#35202,#35203,#35204,#35205,#35206,#35207,#35208,#35209,#35210,
#35211,#35212,#35213,#35214),.UNSPECIFIED.,.F.,.F.,(4,3,3,3,3,3,3,3,3,3,
3,3,3,3,3,3,3,3,3,3,3,3,3,3,3,3,3,3,3,3,3,3,3,3,3,3,3,3,3,3,3,3,3,4),(-2.39814946016205,
-2.31696204062401,-2.29529569174573,-2.2145697251006,-2.15490479499024,
-2.12648768749454,-2.10829922547412,-2.0967829822177,-2.01553459282142,
-1.93371848603571,-1.85215105805855,-1.82342586459833,-1.81332878335441,
-1.80373550349862,-1.73725028421766,-1.65586989316896,-1.5736375593772,
-1.4910414902031,-1.41031007105705,-1.38003578887728,-1.37054045289983,
-1.36256004385421,-1.27951390929298,-1.19605897401236,-1.16811581361891,
-1.08502370215676,-1.00162059508676,-0.950031359376745,-0.926067851441389,
-0.912515239871559,-0.828732202575563,-0.744476327910997,-0.660367724053132,
-0.588906709406608,-0.515293370730782,-0.483087535060108,-0.463174686568405,
-0.454053033116952,-0.370331890792948,-0.285650840288278,-0.200462224975479,
-0.115556068532172,-0.0317686353808436,0.),.UNSPECIFIED.);
#624=B_SPLINE_CURVE_WITH_KNOTS('',3,(#35219,#35220,#35221,#35222,#35223,
#35224,#35225,#35226,#35227,#35228,#35229,#35230,#35231,#35232,#35233,#35234,
#35235,#35236,#35237,#35238,#35239,#35240,#35241,#35242,#35243,#35244,#35245,
#35246,#35247,#35248,#35249,#35250,#35251,#35252,#35253,#35254,#35255,#35256,
#35257,#35258,#35259,#35260,#35261,#35262,#35263,#35264,#35265,#35266,#35267,
#35268,#35269,#35270,#35271,#35272,#35273,#35274,#35275,#35276,#35277,#35278,
#35279,#35280,#35281,#35282,#35283,#35284,#35285,#35286,#35287,#35288,#35289,
#35290,#35291,#35292,#35293,#35294,#35295,#35296,#35297,#35298,#35299,#35300,
#35301,#35302,#35303,#35304,#35305,#35306,#35307,#35308,#35309,#35310,#35311,
#35312,#35313,#35314,#35315,#35316,#35317,#35318,#35319,#35320,#35321,#35322,
#35323,#35324,#35325,#35326,#35327,#35328,#35329,#35330,#35331,#35332,#35333,
#35334,#35335,#35336,#35337,#35338,#35339,#35340,#35341,#35342,#35343,#35344,
#35345,#35346,#35347,#35348),.UNSPECIFIED.,.F.,.F.,(4,3,3,3,3,3,3,3,3,3,
3,3,3,3,3,3,3,3,3,3,3,3,3,3,3,3,3,3,3,3,3,3,3,3,3,3,3,3,3,3,3,3,3,4),(-2.3943990841377,
-2.30957055649357,-2.28423857194396,-2.19921237127506,-2.13667984910918,
-2.1046486142086,-2.08645022202531,-2.07576631330251,-1.99136800229055,
-1.90707270864944,-1.82339088267649,-1.79228121049439,-1.77736473146188,
-1.76769647286273,-1.69895219394807,-1.61556580382811,-1.53168463492449,
-1.44789197014347,-1.36656757293171,-1.3360709239773,-1.3261367157783,-1.31756701043144,
-1.23465419018272,-1.15190857364025,-1.12259438129642,-1.03956979670933,
-0.956697210017908,-0.906629985558681,-0.883172477530608,-0.87009415021638,
-0.788031687387272,-0.705898295573491,-0.624514274873492,-0.556159414344086,
-0.486639487551075,-0.456224519579133,-0.437728905932789,-0.429197413839012,
-0.348523527132435,-0.267263368798083,-0.186163910537152,-0.105687103755617,
-0.0266191312671287,0.),.UNSPECIFIED.);
#625=B_SPLINE_CURVE_WITH_KNOTS('',3,(#35961,#35962,#35963,#35964,#35965,
#35966,#35967,#35968,#35969,#35970,#35971,#35972,#35973,#35974,#35975,#35976),
 .UNSPECIFIED.,.F.,.F.,(4,3,3,3,3,4),(70.2411659442497,70.4688031619064,
70.9650623391029,71.4613215162994,71.9575806934959,72.3613507876847),
 .UNSPECIFIED.);
#626=B_SPLINE_CURVE_WITH_KNOTS('',3,(#35977,#35978,#35979,#35980,#35981,
#35982,#35983,#35984,#35985,#35986,#35987,#35988,#35989,#35990),
 .UNSPECIFIED.,.F.,.F.,(4,1,1,1,1,1,1,1,1,1,1,4),(10.376176187289,10.7799462814777,
11.2762054586742,11.7724646358708,12.2687238130673,12.7649829902638,13.2612421674603,
13.7575013446569,14.2537605218534,14.7500196990499,15.2462788762464,15.707963267949),
 .UNSPECIFIED.);
#627=B_SPLINE_CURVE_WITH_KNOTS('',3,(#35992,#35993,#35994,#35995,#35996,
#35997,#35998,#35999,#36000,#36001,#36002,#36003),.UNSPECIFIED.,.F.,.F.,
(4,1,1,1,1,1,1,1,1,4),(11.6149723878393,12.1112315650359,12.6074907422324,
13.1037499194289,13.6000090966254,14.096268273822,14.5925274510185,15.088786628215,
15.5850458054115,15.707963267949),.UNSPECIFIED.);
#628=B_SPLINE_CURVE_WITH_KNOTS('',3,(#36616,#36617,#36618,#36619,#36620,
#36621,#36622,#36623,#36624,#36625),.UNSPECIFIED.,.F.,.F.,(4,3,3,4),(-74.4388765794786,
-73.9426174022821,-73.4463582250856,-73.2080292590851),.UNSPECIFIED.);
#903=B_SPLINE_SURFACE_WITH_KNOTS('',3,3,((#35349,#35350,#35351,#35352,#35353,
#35354,#35355,#35356,#35357,#35358,#35359,#35360,#35361,#35362,#35363,#35364,
#35365,#35366,#35367,#35368,#35369,#35370,#35371,#35372,#35373,#35374,#35375,
#35376,#35377,#35378,#35379,#35380,#35381,#35382,#35383,#35384,#35385,#35386,
#35387,#35388,#35389,#35390,#35391,#35392,#35393,#35394,#35395,#35396,#35397,
#35398,#35399,#35400,#35401,#35402,#35403,#35404,#35405,#35406,#35407,#35408,
#35409,#35410,#35411,#35412,#35413,#35414,#35415,#35416,#35417,#35418,#35419,
#35420,#35421,#35422,#35423,#35424,#35425,#35426,#35427,#35428,#35429,#35430,
#35431,#35432,#35433,#35434,#35435,#35436,#35437,#35438,#35439,#35440,#35441,
#35442,#35443,#35444,#35445,#35446,#35447,#35448,#35449,#35450,#35451,#35452,
#35453,#35454,#35455,#35456,#35457,#35458,#35459,#35460,#35461,#35462,#35463,
#35464,#35465,#35466,#35467,#35468,#35469,#35470,#35471,#35472,#35473,#35474,
#35475,#35476,#35477,#35478,#35479,#35480,#35481,#35482,#35483,#35484,#35485,
#35486,#35487,#35488,#35489,#35490,#35491,#35492,#35493,#35494,#35495,#35496,
#35497,#35498,#35499,#35500,#35501),(#35502,#35503,#35504,#35505,#35506,
#35507,#35508,#35509,#35510,#35511,#35512,#35513,#35514,#35515,#35516,#35517,
#35518,#35519,#35520,#35521,#35522,#35523,#35524,#35525,#35526,#35527,#35528,
#35529,#35530,#35531,#35532,#35533,#35534,#35535,#35536,#35537,#35538,#35539,
#35540,#35541,#35542,#35543,#35544,#35545,#35546,#35547,#35548,#35549,#35550,
#35551,#35552,#35553,#35554,#35555,#35556,#35557,#35558,#35559,#35560,#35561,
#35562,#35563,#35564,#35565,#35566,#35567,#35568,#35569,#35570,#35571,#35572,
#35573,#35574,#35575,#35576,#35577,#35578,#35579,#35580,#35581,#35582,#35583,
#35584,#35585,#35586,#35587,#35588,#35589,#35590,#35591,#35592,#35593,#35594,
#35595,#35596,#35597,#35598,#35599,#35600,#35601,#35602,#35603,#35604,#35605,
#35606,#35607,#35608,#35609,#35610,#35611,#35612,#35613,#35614,#35615,#35616,
#35617,#35618,#35619,#35620,#35621,#35622,#35623,#35624,#35625,#35626,#35627,
#35628,#35629,#35630,#35631,#35632,#35633,#35634,#35635,#35636,#35637,#35638,
#35639,#35640,#35641,#35642,#35643,#35644,#35645,#35646,#35647,#35648,#35649,
#35650,#35651,#35652,#35653,#35654),(#35655,#35656,#35657,#35658,#35659,
#35660,#35661,#35662,#35663,#35664,#35665,#35666,#35667,#35668,#35669,#35670,
#35671,#35672,#35673,#35674,#35675,#35676,#35677,#35678,#35679,#35680,#35681,
#35682,#35683,#35684,#35685,#35686,#35687,#35688,#35689,#35690,#35691,#35692,
#35693,#35694,#35695,#35696,#35697,#35698,#35699,#35700,#35701,#35702,#35703,
#35704,#35705,#35706,#35707,#35708,#35709,#35710,#35711,#35712,#35713,#35714,
#35715,#35716,#35717,#35718,#35719,#35720,#35721,#35722,#35723,#35724,#35725,
#35726,#35727,#35728,#35729,#35730,#35731,#35732,#35733,#35734,#35735,#35736,
#35737,#35738,#35739,#35740,#35741,#35742,#35743,#35744,#35745,#35746,#35747,
#35748,#35749,#35750,#35751,#35752,#35753,#35754,#35755,#35756,#35757,#35758,
#35759,#35760,#35761,#35762,#35763,#35764,#35765,#35766,#35767,#35768,#35769,
#35770,#35771,#35772,#35773,#35774,#35775,#35776,#35777,#35778,#35779,#35780,
#35781,#35782,#35783,#35784,#35785,#35786,#35787,#35788,#35789,#35790,#35791,
#35792,#35793,#35794,#35795,#35796,#35797,#35798,#35799,#35800,#35801,#35802,
#35803,#35804,#35805,#35806,#35807),(#35808,#35809,#35810,#35811,#35812,
#35813,#35814,#35815,#35816,#35817,#35818,#35819,#35820,#35821,#35822,#35823,
#35824,#35825,#35826,#35827,#35828,#35829,#35830,#35831,#35832,#35833,#35834,
#35835,#35836,#35837,#35838,#35839,#35840,#35841,#35842,#35843,#35844,#35845,
#35846,#35847,#35848,#35849,#35850,#35851,#35852,#35853,#35854,#35855,#35856,
#35857,#35858,#35859,#35860,#35861,#35862,#35863,#35864,#35865,#35866,#35867,
#35868,#35869,#35870,#35871,#35872,#35873,#35874,#35875,#35876,#35877,#35878,
#35879,#35880,#35881,#35882,#35883,#35884,#35885,#35886,#35887,#35888,#35889,
#35890,#35891,#35892,#35893,#35894,#35895,#35896,#35897,#35898,#35899,#35900,
#35901,#35902,#35903,#35904,#35905,#35906,#35907,#35908,#35909,#35910,#35911,
#35912,#35913,#35914,#35915,#35916,#35917,#35918,#35919,#35920,#35921,#35922,
#35923,#35924,#35925,#35926,#35927,#35928,#35929,#35930,#35931,#35932,#35933,
#35934,#35935,#35936,#35937,#35938,#35939,#35940,#35941,#35942,#35943,#35944,
#35945,#35946,#35947,#35948,#35949,#35950,#35951,#35952,#35953,#35954,#35955,
#35956,#35957,#35958,#35959,#35960)),.UNSPECIFIED.,.F.,.F.,.F.,(4,4),(4,
1,1,1,1,1,1,1,1,1,1,1,1,1,1,1,1,1,1,1,1,1,1,1,1,1,1,1,1,1,1,1,1,1,1,1,1,
1,1,1,1,1,1,1,1,1,1,1,1,1,1,1,1,1,1,1,1,1,1,1,1,1,1,1,1,1,1,1,1,1,1,1,1,
1,1,1,1,1,1,1,1,1,1,1,1,1,1,1,1,1,1,1,1,1,1,1,1,1,1,1,1,1,1,1,1,1,1,1,1,
1,1,1,1,1,1,1,1,1,1,1,1,1,1,1,1,1,1,1,1,1,1,1,1,1,1,1,1,1,1,1,1,1,1,1,1,
1,1,1,1,1,4),(0.,0.0991945497494695),(8.2986503954951,8.79490957269163,
9.29116874988815,9.78742792708467,10.2836871042812,10.7799462814777,11.2762054586742,
11.7724646358708,12.2687238130673,12.7649829902638,13.2612421674603,13.7575013446569,
14.2537605218534,14.7500196990499,15.2462788762464,15.742538053443,16.2387972306395,
16.735056407836,17.2313155850325,17.7275747622291,18.2238339394256,18.7200931166221,
19.2163522938186,19.7126114710152,20.2088706482117,20.7051298254082,21.2013890026047,
21.6976481798012,22.1939073569978,22.6901665341943,23.1864257113908,23.6826848885873,
24.1789440657839,24.6752032429804,25.1714624201769,25.6677215973734,26.16398077457,
26.6602399517665,27.156499128963,27.6527583061595,28.1490174833561,28.6452766605526,
29.1415358377491,29.6377950149456,30.1340541921422,30.6303133693387,31.1265725465352,
31.6228317237317,32.1190909009282,32.6153500781248,33.1116092553213,33.6078684325178,
34.1041276097143,34.6003867869109,35.0966459641074,35.5929051413039,36.0891643185004,
36.585423495697,37.0816826728935,37.57794185009,38.0742010272865,38.5704602044831,
39.0667193816796,39.5629785588761,40.0592377360726,40.5554969132692,41.0517560904657,
41.5480152676622,42.0442744448587,42.5405336220552,43.0367927992518,43.5330519764483,
44.0293111536448,44.5255703308413,45.0218295080379,45.5180886852344,46.0143478624309,
46.5106070396274,47.006866216824,47.5031253940205,47.999384571217,48.4956437484135,
48.9919029256101,49.4881621028066,49.9844212800031,50.4806804571996,50.9769396343962,
51.4731988115927,51.9694579887892,52.4657171659857,52.9619763431823,53.4582355203788,
53.9544946975753,54.4507538747718,54.9470130519683,55.4432722291649,55.9395314063614,
56.4357905835579,56.9320497607544,57.428308937951,57.9245681151475,58.420827292344,
58.9170864695405,59.4133456467371,59.9096048239336,60.4058640011301,60.9021231783266,
61.3983823555232,61.8946415327197,62.3909007099162,62.8871598871127,63.3834190643093,
63.8796782415058,64.3759374187023,64.8721965958988,65.3684557730953,65.8647149502919,
66.3609741274884,66.8572333046849,67.3534924818814,67.849751659078,68.3460108362745,
68.842270013471,69.3385291906675,69.8347883678641,70.3310475450606,70.8273067222571,
71.3235658994536,71.8198250766501,72.3160842538467,72.8123434310432,73.3086026082397,
73.8048617854362,74.3011209626328,74.7973801398293,75.2936393170258,75.7898984942223,
76.2861576714189,76.7824168486154,77.2786760258119,77.7749352030084,78.271194380205,
78.7674535574015,79.263712734598,79.7599719117945,80.2562310889911,80.7524902661876,
81.2487494433841,81.7450086205806,82.2412677977772,82.7375269749737),
 .UNSPECIFIED.);
#904=B_SPLINE_SURFACE_WITH_KNOTS('',3,3,((#36004,#36005,#36006,#36007,#36008,
#36009,#36010,#36011,#36012,#36013,#36014,#36015,#36016,#36017,#36018,#36019,
#36020,#36021,#36022,#36023,#36024,#36025,#36026,#36027,#36028,#36029,#36030,
#36031,#36032,#36033,#36034,#36035,#36036,#36037,#36038,#36039,#36040,#36041,
#36042,#36043,#36044,#36045,#36046,#36047,#36048,#36049,#36050,#36051,#36052,
#36053,#36054,#36055,#36056,#36057,#36058,#36059,#36060,#36061,#36062,#36063,
#36064,#36065,#36066,#36067,#36068,#36069,#36070,#36071,#36072,#36073,#36074,
#36075,#36076,#36077,#36078,#36079,#36080,#36081,#36082,#36083,#36084,#36085,
#36086,#36087,#36088,#36089,#36090,#36091,#36092,#36093,#36094,#36095,#36096,
#36097,#36098,#36099,#36100,#36101,#36102,#36103,#36104,#36105,#36106,#36107,
#36108,#36109,#36110,#36111,#36112,#36113,#36114,#36115,#36116,#36117,#36118,
#36119,#36120,#36121,#36122,#36123,#36124,#36125,#36126,#36127,#36128,#36129,
#36130,#36131,#36132,#36133,#36134,#36135,#36136,#36137,#36138,#36139,#36140,
#36141,#36142,#36143,#36144,#36145,#36146,#36147,#36148,#36149,#36150,#36151,
#36152,#36153,#36154,#36155,#36156),(#36157,#36158,#36159,#36160,#36161,
#36162,#36163,#36164,#36165,#36166,#36167,#36168,#36169,#36170,#36171,#36172,
#36173,#36174,#36175,#36176,#36177,#36178,#36179,#36180,#36181,#36182,#36183,
#36184,#36185,#36186,#36187,#36188,#36189,#36190,#36191,#36192,#36193,#36194,
#36195,#36196,#36197,#36198,#36199,#36200,#36201,#36202,#36203,#36204,#36205,
#36206,#36207,#36208,#36209,#36210,#36211,#36212,#36213,#36214,#36215,#36216,
#36217,#36218,#36219,#36220,#36221,#36222,#36223,#36224,#36225,#36226,#36227,
#36228,#36229,#36230,#36231,#36232,#36233,#36234,#36235,#36236,#36237,#36238,
#36239,#36240,#36241,#36242,#36243,#36244,#36245,#36246,#36247,#36248,#36249,
#36250,#36251,#36252,#36253,#36254,#36255,#36256,#36257,#36258,#36259,#36260,
#36261,#36262,#36263,#36264,#36265,#36266,#36267,#36268,#36269,#36270,#36271,
#36272,#36273,#36274,#36275,#36276,#36277,#36278,#36279,#36280,#36281,#36282,
#36283,#36284,#36285,#36286,#36287,#36288,#36289,#36290,#36291,#36292,#36293,
#36294,#36295,#36296,#36297,#36298,#36299,#36300,#36301,#36302,#36303,#36304,
#36305,#36306,#36307,#36308,#36309),(#36310,#36311,#36312,#36313,#36314,
#36315,#36316,#36317,#36318,#36319,#36320,#36321,#36322,#36323,#36324,#36325,
#36326,#36327,#36328,#36329,#36330,#36331,#36332,#36333,#36334,#36335,#36336,
#36337,#36338,#36339,#36340,#36341,#36342,#36343,#36344,#36345,#36346,#36347,
#36348,#36349,#36350,#36351,#36352,#36353,#36354,#36355,#36356,#36357,#36358,
#36359,#36360,#36361,#36362,#36363,#36364,#36365,#36366,#36367,#36368,#36369,
#36370,#36371,#36372,#36373,#36374,#36375,#36376,#36377,#36378,#36379,#36380,
#36381,#36382,#36383,#36384,#36385,#36386,#36387,#36388,#36389,#36390,#36391,
#36392,#36393,#36394,#36395,#36396,#36397,#36398,#36399,#36400,#36401,#36402,
#36403,#36404,#36405,#36406,#36407,#36408,#36409,#36410,#36411,#36412,#36413,
#36414,#36415,#36416,#36417,#36418,#36419,#36420,#36421,#36422,#36423,#36424,
#36425,#36426,#36427,#36428,#36429,#36430,#36431,#36432,#36433,#36434,#36435,
#36436,#36437,#36438,#36439,#36440,#36441,#36442,#36443,#36444,#36445,#36446,
#36447,#36448,#36449,#36450,#36451,#36452,#36453,#36454,#36455,#36456,#36457,
#36458,#36459,#36460,#36461,#36462),(#36463,#36464,#36465,#36466,#36467,
#36468,#36469,#36470,#36471,#36472,#36473,#36474,#36475,#36476,#36477,#36478,
#36479,#36480,#36481,#36482,#36483,#36484,#36485,#36486,#36487,#36488,#36489,
#36490,#36491,#36492,#36493,#36494,#36495,#36496,#36497,#36498,#36499,#36500,
#36501,#36502,#36503,#36504,#36505,#36506,#36507,#36508,#36509,#36510,#36511,
#36512,#36513,#36514,#36515,#36516,#36517,#36518,#36519,#36520,#36521,#36522,
#36523,#36524,#36525,#36526,#36527,#36528,#36529,#36530,#36531,#36532,#36533,
#36534,#36535,#36536,#36537,#36538,#36539,#36540,#36541,#36542,#36543,#36544,
#36545,#36546,#36547,#36548,#36549,#36550,#36551,#36552,#36553,#36554,#36555,
#36556,#36557,#36558,#36559,#36560,#36561,#36562,#36563,#36564,#36565,#36566,
#36567,#36568,#36569,#36570,#36571,#36572,#36573,#36574,#36575,#36576,#36577,
#36578,#36579,#36580,#36581,#36582,#36583,#36584,#36585,#36586,#36587,#36588,
#36589,#36590,#36591,#36592,#36593,#36594,#36595,#36596,#36597,#36598,#36599,
#36600,#36601,#36602,#36603,#36604,#36605,#36606,#36607,#36608,#36609,#36610,
#36611,#36612,#36613,#36614,#36615)),.UNSPECIFIED.,.F.,.F.,.F.,(4,4),(4,
1,1,1,1,1,1,1,1,1,1,1,1,1,1,1,1,1,1,1,1,1,1,1,1,1,1,1,1,1,1,1,1,1,1,1,1,
1,1,1,1,1,1,1,1,1,1,1,1,1,1,1,1,1,1,1,1,1,1,1,1,1,1,1,1,1,1,1,1,1,1,1,1,
1,1,1,1,1,1,1,1,1,1,1,1,1,1,1,1,1,1,1,1,1,1,1,1,1,1,1,1,1,1,1,1,1,1,1,1,
1,1,1,1,1,1,1,1,1,1,1,1,1,1,1,1,1,1,1,1,1,1,1,1,1,1,1,1,1,1,1,1,1,1,1,1,
1,1,1,1,1,4),(0.,0.0991945497494695),(11.6149723878393,12.1112315650359,
12.6074907422324,13.1037499194289,13.6000090966254,14.096268273822,14.5925274510185,
15.088786628215,15.5850458054115,16.0813049826081,16.5775641598046,17.0738233370011,
17.5700825141976,18.0663416913942,18.5626008685907,19.0588600457872,19.5551192229837,
20.0513784001803,20.5476375773768,21.0438967545733,21.5401559317698,22.0364151089663,
22.5326742861629,23.0289334633594,23.5251926405559,24.0214518177524,24.517710994949,
25.0139701721455,25.510229349342,26.0064885265385,26.5027477037351,26.9990068809316,
27.4952660581281,27.9915252353246,28.4877844125212,28.9840435897177,29.4803027669142,
29.9765619441107,30.4728211213073,30.9690802985038,31.4653394757003,31.9615986528968,
32.4578578300934,32.9541170072899,33.4503761844864,33.9466353616829,34.4428945388795,
34.939153716076,35.4354128932725,35.931672070469,36.4279312476656,36.9241904248621,
37.4204496020586,37.9167087792551,38.4129679564517,38.9092271336482,39.4054863108447,
39.9017454880412,40.3980046652377,40.8942638424343,41.3905230196308,41.8867821968273,
42.3830413740238,42.8793005512204,43.3755597284169,43.8718189056134,44.36807808281,
44.8643372600065,45.360596437203,45.8568556143995,46.353114791596,46.8493739687926,
47.3456331459891,47.8418923231856,48.3381515003821,48.8344106775787,49.3306698547752,
49.8269290319717,50.3231882091682,50.8194473863648,51.3157065635613,51.8119657407578,
52.3082249179543,52.8044840951509,53.3007432723474,53.7970024495439,54.2932616267404,
54.789520803937,55.2857799811335,55.78203915833,56.2782983355265,56.7745575127231,
57.2708166899196,57.7670758671161,58.2633350443126,58.7595942215092,59.2558533987057,
59.7521125759022,60.2483717530987,60.7446309302953,61.2408901074918,61.7371492846883,
62.2334084618848,62.7296676390814,63.2259268162779,63.7221859934744,64.2184451706709,
64.7147043478674,65.210963525064,65.7072227022605,66.203481879457,66.6997410566536,
67.1960002338501,67.6922594110466,68.1885185882431,68.6847777654396,69.1810369426362,
69.6772961198327,70.1735552970292,70.6698144742257,71.1660736514223,71.6623328286188,
72.1585920058153,72.6548511830118,73.1511103602084,73.6473695374049,74.1436287146014,
74.6398878917979,75.1361470689945,75.632406246191,76.1286654233875,76.624924600584,
77.1211837777806,77.6174429549771,78.1137021321736,78.6099613093701,79.1062204865667,
79.6024796637632,80.0987388409597,80.5949980181562,81.0912571953528,81.5875163725493,
82.0837755497458,82.5800347269423,83.0762939041389,83.5725530813354,84.0688122585319,
84.5650714357284,85.061330612925,85.5575897901215,86.053848967318),
 .UNSPECIFIED.);
#974=FACE_BOUND('',#3271,.T.);
#975=FACE_BOUND('',#3281,.T.);
#976=FACE_BOUND('',#3285,.T.);
#977=FACE_BOUND('',#3288,.T.);
#978=FACE_BOUND('',#3291,.T.);
#1219=PLANE('',#17312);
#1220=PLANE('',#17319);
#1221=PLANE('',#17328);
#1222=PLANE('',#17333);
#1223=PLANE('',#17337);
#1224=PLANE('',#17341);
#1689=CYLINDRICAL_SURFACE('',#17280,11.925);
#1690=CYLINDRICAL_SURFACE('',#17282,11.925);
#1691=CYLINDRICAL_SURFACE('',#17283,11.925);
#1692=CYLINDRICAL_SURFACE('',#17284,11.925);
#1693=CYLINDRICAL_SURFACE('',#17285,11.925);
#1694=CYLINDRICAL_SURFACE('',#17286,11.925);
#1695=CYLINDRICAL_SURFACE('',#17287,11.925);
#1696=CYLINDRICAL_SURFACE('',#17288,11.925);
#1697=CYLINDRICAL_SURFACE('',#17289,11.925);
#1698=CYLINDRICAL_SURFACE('',#17290,11.925);
#1699=CYLINDRICAL_SURFACE('',#17291,11.925);
#1700=CYLINDRICAL_SURFACE('',#17292,11.925);
#1701=CYLINDRICAL_SURFACE('',#17293,11.06595);
#1702=CYLINDRICAL_SURFACE('',#17295,11.06595);
#1703=CYLINDRICAL_SURFACE('',#17296,11.06595);
#1704=CYLINDRICAL_SURFACE('',#17297,11.06595);
#1705=CYLINDRICAL_SURFACE('',#17298,11.06595);
#1706=CYLINDRICAL_SURFACE('',#17299,11.06595);
#1707=CYLINDRICAL_SURFACE('',#17300,11.06595);
#1708=CYLINDRICAL_SURFACE('',#17301,11.06595);
#1709=CYLINDRICAL_SURFACE('',#17302,11.06595);
#1710=CYLINDRICAL_SURFACE('',#17303,11.06595);
#1711=CYLINDRICAL_SURFACE('',#17304,11.06595);
#1712=CYLINDRICAL_SURFACE('',#17317,23.);
#1713=CYLINDRICAL_SURFACE('',#17322,11.06595);
#1714=CYLINDRICAL_SURFACE('',#17323,11.925);
#1715=CYLINDRICAL_SURFACE('',#17325,16.55);
#1716=CYLINDRICAL_SURFACE('',#17335,5.05);
#1717=CYLINDRICAL_SURFACE('',#17339,17.5);
#2236=FACE_OUTER_BOUND('',#3245,.T.);
#2237=FACE_OUTER_BOUND('',#3246,.T.);
#2238=FACE_OUTER_BOUND('',#3247,.T.);
#2239=FACE_OUTER_BOUND('',#3248,.T.);
#2240=FACE_OUTER_BOUND('',#3249,.T.);
#2241=FACE_OUTER_BOUND('',#3250,.T.);
#2242=FACE_OUTER_BOUND('',#3251,.T.);
#2243=FACE_OUTER_BOUND('',#3252,.T.);
#2244=FACE_OUTER_BOUND('',#3253,.T.);
#2245=FACE_OUTER_BOUND('',#3254,.T.);
#2246=FACE_OUTER_BOUND('',#3255,.T.);
#2247=FACE_OUTER_BOUND('',#3256,.T.);
#2248=FACE_OUTER_BOUND('',#3257,.T.);
#2249=FACE_OUTER_BOUND('',#3258,.T.);
#2250=FACE_OUTER_BOUND('',#3259,.T.);
#2251=FACE_OUTER_BOUND('',#3260,.T.);
#2252=FACE_OUTER_BOUND('',#3261,.T.);
#2253=FACE_OUTER_BOUND('',#3262,.T.);
#2254=FACE_OUTER_BOUND('',#3263,.T.);
#2255=FACE_OUTER_BOUND('',#3264,.T.);
#2256=FACE_OUTER_BOUND('',#3265,.T.);
#2257=FACE_OUTER_BOUND('',#3266,.T.);
#2258=FACE_OUTER_BOUND('',#3267,.T.);
#2259=FACE_OUTER_BOUND('',#3268,.T.);
#2260=FACE_OUTER_BOUND('',#3269,.T.);
#2261=FACE_OUTER_BOUND('',#3270,.T.);
#2262=FACE_OUTER_BOUND('',#3272,.T.);
#2263=FACE_OUTER_BOUND('',#3273,.T.);
#2264=FACE_OUTER_BOUND('',#3274,.T.);
#2265=FACE_OUTER_BOUND('',#3275,.T.);
#2266=FACE_OUTER_BOUND('',#3276,.T.);
#2267=FACE_OUTER_BOUND('',#3277,.T.);
#2268=FACE_OUTER_BOUND('',#3278,.T.);
#2269=FACE_OUTER_BOUND('',#3279,.T.);
#2270=FACE_OUTER_BOUND('',#3280,.T.);
#2271=FACE_OUTER_BOUND('',#3282,.T.);
#2272=FACE_OUTER_BOUND('',#3283,.T.);
#2273=FACE_OUTER_BOUND('',#3284,.T.);
#2274=FACE_OUTER_BOUND('',#3286,.T.);
#2275=FACE_OUTER_BOUND('',#3287,.T.);
#2276=FACE_OUTER_BOUND('',#3289,.T.);
#2277=FACE_OUTER_BOUND('',#3290,.T.);
#3245=EDGE_LOOP('',(#12868,#12869,#12870,#12871));
#3246=EDGE_LOOP('',(#12872,#12873,#12874,#12875));
#3247=EDGE_LOOP('',(#12876,#12877,#12878,#12879));
#3248=EDGE_LOOP('',(#12880,#12881,#12882,#12883));
#3249=EDGE_LOOP('',(#12884,#12885,#12886,#12887));
#3250=EDGE_LOOP('',(#12888,#12889,#12890,#12891));
#3251=EDGE_LOOP('',(#12892,#12893,#12894,#12895));
#3252=EDGE_LOOP('',(#12896,#12897,#12898,#12899));
#3253=EDGE_LOOP('',(#12900,#12901,#12902,#12903));
#3254=EDGE_LOOP('',(#12904,#12905,#12906,#12907));
#3255=EDGE_LOOP('',(#12908,#12909,#12910,#12911));
#3256=EDGE_LOOP('',(#12912,#12913,#12914,#12915));
#3257=EDGE_LOOP('',(#12916,#12917,#12918,#12919));
#3258=EDGE_LOOP('',(#12920,#12921,#12922,#12923));
#3259=EDGE_LOOP('',(#12924,#12925,#12926,#12927));
#3260=EDGE_LOOP('',(#12928,#12929,#12930,#12931));
#3261=EDGE_LOOP('',(#12932,#12933,#12934,#12935));
#3262=EDGE_LOOP('',(#12936,#12937,#12938,#12939));
#3263=EDGE_LOOP('',(#12940,#12941,#12942,#12943));
#3264=EDGE_LOOP('',(#12944,#12945,#12946,#12947));
#3265=EDGE_LOOP('',(#12948,#12949,#12950,#12951));
#3266=EDGE_LOOP('',(#12952,#12953,#12954,#12955));
#3267=EDGE_LOOP('',(#12956,#12957,#12958,#12959));
#3268=EDGE_LOOP('',(#12960,#12961,#12962,#12963,#12964));
#3269=EDGE_LOOP('',(#12965,#12966,#12967,#12968,#12969,#12970));
#3270=EDGE_LOOP('',(#12971));
#3271=EDGE_LOOP('',(#12972,#12973,#12974,#12975));
#3272=EDGE_LOOP('',(#12976,#12977,#12978,#12979,#12980,#12981));
#3273=EDGE_LOOP('',(#12982,#12983,#12984,#12985,#12986));
#3274=EDGE_LOOP('',(#12987,#12988,#12989,#12990,#12991));
#3275=EDGE_LOOP('',(#12992,#12993,#12994,#12995,#12996,#12997,#12998,#12999,
#13000,#13001,#13002,#13003,#13004,#13005,#13006,#13007,#13008,#13009,#13010,
#13011,#13012,#13013,#13014,#13015,#13016,#13017,#13018));
#3276=EDGE_LOOP('',(#13019,#13020,#13021,#13022));
#3277=EDGE_LOOP('',(#13023,#13024,#13025,#13026,#13027,#13028,#13029,#13030,
#13031,#13032,#13033,#13034,#13035,#13036,#13037,#13038,#13039,#13040,#13041,
#13042,#13043,#13044,#13045,#13046,#13047,#13048,#13049));
#3278=EDGE_LOOP('',(#13050,#13051,#13052,#13053));
#3279=EDGE_LOOP('',(#13054,#13055,#13056,#13057));
#3280=EDGE_LOOP('',(#13058));
#3281=EDGE_LOOP('',(#13059));
#3282=EDGE_LOOP('',(#13060,#13061,#13062,#13063));
#3283=EDGE_LOOP('',(#13064,#13065,#13066,#13067,#13068,#13069));
#3284=EDGE_LOOP('',(#13070));
#3285=EDGE_LOOP('',(#13071));
#3286=EDGE_LOOP('',(#13072,#13073,#13074,#13075));
#3287=EDGE_LOOP('',(#13076));
#3288=EDGE_LOOP('',(#13077));
#3289=EDGE_LOOP('',(#13078,#13079,#13080,#13081));
#3290=EDGE_LOOP('',(#13082));
#3291=EDGE_LOOP('',(#13083));
#4421=LINE('',#33392,#5732);
#4422=LINE('',#33425,#5733);
#4423=LINE('',#33509,#5734);
#4424=LINE('',#33599,#5735);
#4425=LINE('',#33689,#5736);
#4426=LINE('',#33773,#5737);
#4427=LINE('',#33863,#5738);
#4428=LINE('',#33953,#5739);
#4429=LINE('',#34037,#5740);
#4430=LINE('',#34127,#5741);
#4431=LINE('',#34217,#5742);
#4432=LINE('',#34301,#5743);
#4433=LINE('',#34391,#5744);
#4434=LINE('',#34425,#5745);
#4435=LINE('',#34462,#5746);
#4436=LINE('',#34499,#5747);
#4437=LINE('',#34537,#5748);
#4438=LINE('',#34574,#5749);
#4439=LINE('',#34611,#5750);
#4440=LINE('',#34649,#5751);
#4441=LINE('',#34686,#5752);
#4442=LINE('',#34723,#5753);
#4443=LINE('',#34761,#5754);
#4444=LINE('',#34799,#5755);
#4445=LINE('',#34805,#5756);
#4446=LINE('',#35075,#5757);
#4447=LINE('',#35081,#5758);
#4448=LINE('',#36632,#5759);
#4449=LINE('',#36638,#5760);
#4450=LINE('',#36642,#5761);
#4451=LINE('',#36648,#5762);
#4452=LINE('',#36655,#5763);
#5732=VECTOR('',#19704,12.);
#5733=VECTOR('',#19709,12.);
#5734=VECTOR('',#19712,12.);
#5735=VECTOR('',#19715,12.);
#5736=VECTOR('',#19718,12.);
#5737=VECTOR('',#19721,12.);
#5738=VECTOR('',#19724,12.);
#5739=VECTOR('',#19727,12.);
#5740=VECTOR('',#19730,12.);
#5741=VECTOR('',#19733,12.);
#5742=VECTOR('',#19736,12.);
#5743=VECTOR('',#19739,12.);
#5744=VECTOR('',#19742,11.06595);
#5745=VECTOR('',#19747,11.06595);
#5746=VECTOR('',#19750,11.06595);
#5747=VECTOR('',#19753,11.06595);
#5748=VECTOR('',#19756,11.06595);
#5749=VECTOR('',#19759,11.06595);
#5750=VECTOR('',#19762,11.06595);
#5751=VECTOR('',#19765,11.06595);
#5752=VECTOR('',#19768,11.06595);
#5753=VECTOR('',#19771,11.06595);
#5754=VECTOR('',#19774,11.06595);
#5755=VECTOR('',#19779,14.9061737618886);
#5756=VECTOR('',#19786,19.);
#5757=VECTOR('',#19797,22.8438262381114);
#5758=VECTOR('',#19804,23.);
#5759=VECTOR('',#19823,16.55);
#5760=VECTOR('',#19832,22.6);
#5761=VECTOR('',#19837,11.6);
#5762=VECTOR('',#19844,5.05);
#5763=VECTOR('',#19853,17.5);
#6685=CIRCLE('',#17281,11.925);
#6686=CIRCLE('',#17294,11.06595);
#6687=CIRCLE('',#17306,14.5);
#6688=CIRCLE('',#17307,15.3123475237772);
#6689=CIRCLE('',#17308,15.3123475237772);
#6690=CIRCLE('',#17310,22.6876524762228);
#6691=CIRCLE('',#17311,22.6876524762228);
#6692=CIRCLE('',#17313,11.06595);
#6693=CIRCLE('',#17315,23.);
#6694=CIRCLE('',#17316,23.);
#6695=CIRCLE('',#17318,23.);
#6696=CIRCLE('',#17320,11.925);
#6697=CIRCLE('',#17321,11.925);
#6698=CIRCLE('',#17324,11.925);
#6699=CIRCLE('',#17326,16.55);
#6700=CIRCLE('',#17327,16.55);
#6701=CIRCLE('',#17329,22.2);
#6702=CIRCLE('',#17332,11.2);
#6703=CIRCLE('',#17334,5.05);
#6704=CIRCLE('',#17336,5.05);
#6705=CIRCLE('',#17338,17.5);
#6706=CIRCLE('',#17340,17.5);
#7618=VERTEX_POINT('',#33390);
#7619=VERTEX_POINT('',#33391);
#7620=VERTEX_POINT('',#33393);
#7621=VERTEX_POINT('',#33410);
#7622=VERTEX_POINT('',#33423);
#7623=VERTEX_POINT('',#33424);
#7624=VERTEX_POINT('',#33507);
#7625=VERTEX_POINT('',#33508);
#7626=VERTEX_POINT('',#33597);
#7627=VERTEX_POINT('',#33598);
#7628=VERTEX_POINT('',#33687);
#7629=VERTEX_POINT('',#33688);
#7630=VERTEX_POINT('',#33771);
#7631=VERTEX_POINT('',#33772);
#7632=VERTEX_POINT('',#33861);
#7633=VERTEX_POINT('',#33862);
#7634=VERTEX_POINT('',#33951);
#7635=VERTEX_POINT('',#33952);
#7636=VERTEX_POINT('',#34035);
#7637=VERTEX_POINT('',#34036);
#7638=VERTEX_POINT('',#34125);
#7639=VERTEX_POINT('',#34126);
#7640=VERTEX_POINT('',#34215);
#7641=VERTEX_POINT('',#34216);
#7642=VERTEX_POINT('',#34299);
#7643=VERTEX_POINT('',#34300);
#7644=VERTEX_POINT('',#34389);
#7645=VERTEX_POINT('',#34390);
#7646=VERTEX_POINT('',#34392);
#7647=VERTEX_POINT('',#34408);
#7648=VERTEX_POINT('',#34423);
#7649=VERTEX_POINT('',#34424);
#7650=VERTEX_POINT('',#34460);
#7651=VERTEX_POINT('',#34461);
#7652=VERTEX_POINT('',#34497);
#7653=VERTEX_POINT('',#34498);
#7654=VERTEX_POINT('',#34535);
#7655=VERTEX_POINT('',#34536);
#7656=VERTEX_POINT('',#34572);
#7657=VERTEX_POINT('',#34573);
#7658=VERTEX_POINT('',#34609);
#7659=VERTEX_POINT('',#34610);
#7660=VERTEX_POINT('',#34647);
#7661=VERTEX_POINT('',#34648);
#7662=VERTEX_POINT('',#34684);
#7663=VERTEX_POINT('',#34685);
#7664=VERTEX_POINT('',#34721);
#7665=VERTEX_POINT('',#34722);
#7666=VERTEX_POINT('',#34759);
#7667=VERTEX_POINT('',#34760);
#7668=VERTEX_POINT('',#34796);
#7669=VERTEX_POINT('',#34798);
#7670=VERTEX_POINT('',#34800);
#7671=VERTEX_POINT('',#34804);
#7672=VERTEX_POINT('',#34806);
#7673=VERTEX_POINT('',#34810);
#7674=VERTEX_POINT('',#34941);
#7675=VERTEX_POINT('',#35074);
#7676=VERTEX_POINT('',#35076);
#7677=VERTEX_POINT('',#35080);
#7678=VERTEX_POINT('',#35084);
#7679=VERTEX_POINT('',#35215);
#7680=VERTEX_POINT('',#35217);
#7681=VERTEX_POINT('',#36629);
#7682=VERTEX_POINT('',#36631);
#7683=VERTEX_POINT('',#36635);
#7684=VERTEX_POINT('',#36640);
#7685=VERTEX_POINT('',#36644);
#7686=VERTEX_POINT('',#36647);
#7687=VERTEX_POINT('',#36651);
#7688=VERTEX_POINT('',#36654);
#9497=EDGE_CURVE('',#7618,#7619,#4421,.T.);
#9498=EDGE_CURVE('',#7618,#7620,#575,.T.);
#9499=EDGE_CURVE('',#7620,#7621,#6685,.F.);
#9500=EDGE_CURVE('',#7621,#7619,#576,.T.);
#9501=EDGE_CURVE('',#7622,#7623,#4422,.T.);
#9502=EDGE_CURVE('',#7622,#7618,#577,.T.);
#9503=EDGE_CURVE('',#7619,#7623,#578,.T.);
#9504=EDGE_CURVE('',#7624,#7625,#4423,.T.);
#9505=EDGE_CURVE('',#7624,#7622,#579,.T.);
#9506=EDGE_CURVE('',#7623,#7625,#580,.T.);
#9507=EDGE_CURVE('',#7626,#7627,#4424,.T.);
#9508=EDGE_CURVE('',#7626,#7624,#581,.T.);
#9509=EDGE_CURVE('',#7625,#7627,#582,.T.);
#9510=EDGE_CURVE('',#7628,#7629,#4425,.T.);
#9511=EDGE_CURVE('',#7628,#7626,#583,.T.);
#9512=EDGE_CURVE('',#7627,#7629,#584,.T.);
#9513=EDGE_CURVE('',#7630,#7631,#4426,.T.);
#9514=EDGE_CURVE('',#7630,#7628,#585,.T.);
#9515=EDGE_CURVE('',#7629,#7631,#586,.T.);
#9516=EDGE_CURVE('',#7632,#7633,#4427,.T.);
#9517=EDGE_CURVE('',#7632,#7630,#587,.T.);
#9518=EDGE_CURVE('',#7631,#7633,#588,.T.);
#9519=EDGE_CURVE('',#7634,#7635,#4428,.T.);
#9520=EDGE_CURVE('',#7634,#7632,#589,.T.);
#9521=EDGE_CURVE('',#7633,#7635,#590,.T.);
#9522=EDGE_CURVE('',#7636,#7637,#4429,.T.);
#9523=EDGE_CURVE('',#7636,#7634,#591,.T.);
#9524=EDGE_CURVE('',#7635,#7637,#592,.T.);
#9525=EDGE_CURVE('',#7638,#7639,#4430,.T.);
#9526=EDGE_CURVE('',#7638,#7636,#593,.T.);
#9527=EDGE_CURVE('',#7637,#7639,#594,.T.);
#9528=EDGE_CURVE('',#7640,#7641,#4431,.T.);
#9529=EDGE_CURVE('',#7640,#7638,#595,.T.);
#9530=EDGE_CURVE('',#7639,#7641,#596,.T.);
#9531=EDGE_CURVE('',#7642,#7643,#4432,.T.);
#9532=EDGE_CURVE('',#7642,#7640,#597,.T.);
#9533=EDGE_CURVE('',#7641,#7643,#598,.T.);
#9534=EDGE_CURVE('',#7644,#7645,#4433,.T.);
#9535=EDGE_CURVE('',#7644,#7646,#599,.T.);
#9536=EDGE_CURVE('',#7647,#7646,#6686,.T.);
#9537=EDGE_CURVE('',#7645,#7647,#600,.T.);
#9538=EDGE_CURVE('',#7648,#7649,#4434,.T.);
#9539=EDGE_CURVE('',#7648,#7644,#601,.T.);
#9540=EDGE_CURVE('',#7649,#7645,#602,.T.);
#9541=EDGE_CURVE('',#7650,#7651,#4435,.T.);
#9542=EDGE_CURVE('',#7650,#7648,#603,.T.);
#9543=EDGE_CURVE('',#7651,#7649,#604,.T.);
#9544=EDGE_CURVE('',#7652,#7653,#4436,.T.);
#9545=EDGE_CURVE('',#7652,#7650,#605,.T.);
#9546=EDGE_CURVE('',#7653,#7651,#606,.T.);
#9547=EDGE_CURVE('',#7654,#7655,#4437,.T.);
#9548=EDGE_CURVE('',#7654,#7652,#607,.T.);
#9549=EDGE_CURVE('',#7655,#7653,#608,.T.);
#9550=EDGE_CURVE('',#7656,#7657,#4438,.T.);
#9551=EDGE_CURVE('',#7656,#7654,#609,.T.);
#9552=EDGE_CURVE('',#7657,#7655,#610,.T.);
#9553=EDGE_CURVE('',#7658,#7659,#4439,.T.);
#9554=EDGE_CURVE('',#7658,#7656,#611,.T.);
#9555=EDGE_CURVE('',#7659,#7657,#612,.T.);
#9556=EDGE_CURVE('',#7660,#7661,#4440,.T.);
#9557=EDGE_CURVE('',#7660,#7658,#613,.T.);
#9558=EDGE_CURVE('',#7661,#7659,#614,.T.);
#9559=EDGE_CURVE('',#7662,#7663,#4441,.T.);
#9560=EDGE_CURVE('',#7662,#7660,#615,.T.);
#9561=EDGE_CURVE('',#7663,#7661,#616,.T.);
#9562=EDGE_CURVE('',#7664,#7665,#4442,.T.);
#9563=EDGE_CURVE('',#7664,#7662,#617,.T.);
#9564=EDGE_CURVE('',#7665,#7663,#618,.T.);
#9565=EDGE_CURVE('',#7666,#7667,#4443,.T.);
#9566=EDGE_CURVE('',#7666,#7664,#619,.T.);
#9567=EDGE_CURVE('',#7667,#7665,#620,.T.);
#9568=EDGE_CURVE('',#7668,#7668,#6687,.T.);
#9569=EDGE_CURVE('',#7668,#7669,#4444,.T.);
#9570=EDGE_CURVE('',#7669,#7670,#6688,.T.);
#9571=EDGE_CURVE('',#7670,#7669,#6689,.T.);
#9572=EDGE_CURVE('',#7670,#7671,#4445,.T.);
#9573=EDGE_CURVE('',#7672,#7671,#6690,.T.);
#9574=EDGE_CURVE('',#7671,#7672,#6691,.T.);
#9575=EDGE_CURVE('',#7620,#7673,#621,.T.);
#9576=EDGE_CURVE('',#7673,#7674,#6692,.T.);
#9577=EDGE_CURVE('',#7674,#7621,#622,.T.);
#9578=EDGE_CURVE('',#7672,#7675,#4446,.T.);
#9579=EDGE_CURVE('',#7675,#7676,#6693,.T.);
#9580=EDGE_CURVE('',#7676,#7675,#6694,.T.);
#9581=EDGE_CURVE('',#7676,#7677,#4447,.T.);
#9582=EDGE_CURVE('',#7677,#7677,#6695,.T.);
#9583=EDGE_CURVE('',#7646,#7678,#623,.T.);
#9584=EDGE_CURVE('',#7679,#7678,#6696,.F.);
#9585=EDGE_CURVE('',#7680,#7679,#6697,.F.);
#9586=EDGE_CURVE('',#7680,#7647,#624,.T.);
#9587=EDGE_CURVE('',#7643,#7680,#625,.T.);
#9588=EDGE_CURVE('',#7674,#7667,#626,.T.);
#9589=EDGE_CURVE('',#7673,#7666,#627,.T.);
#9590=EDGE_CURVE('',#7678,#7642,#628,.T.);
#9591=EDGE_CURVE('',#7678,#7680,#6698,.F.);
#9592=EDGE_CURVE('',#7681,#7681,#6699,.T.);
#9593=EDGE_CURVE('',#7681,#7682,#4448,.T.);
#9594=EDGE_CURVE('',#7682,#7682,#6700,.T.);
#9595=EDGE_CURVE('',#7683,#7683,#6701,.T.);
#9596=EDGE_CURVE('',#7677,#7683,#4449,.T.);
#9597=EDGE_CURVE('',#7684,#7684,#6702,.T.);
#9598=EDGE_CURVE('',#7684,#7679,#4450,.T.);
#9599=EDGE_CURVE('',#7685,#7685,#6703,.T.);
#9600=EDGE_CURVE('',#7685,#7686,#4451,.T.);
#9601=EDGE_CURVE('',#7686,#7686,#6704,.T.);
#9602=EDGE_CURVE('',#7687,#7687,#6705,.T.);
#9603=EDGE_CURVE('',#7687,#7688,#4452,.T.);
#9604=EDGE_CURVE('',#7688,#7688,#6706,.T.);
#12868=ORIENTED_EDGE('',*,*,#9497,.F.);
#12869=ORIENTED_EDGE('',*,*,#9498,.T.);
#12870=ORIENTED_EDGE('',*,*,#9499,.T.);
#12871=ORIENTED_EDGE('',*,*,#9500,.T.);
#12872=ORIENTED_EDGE('',*,*,#9501,.F.);
#12873=ORIENTED_EDGE('',*,*,#9502,.T.);
#12874=ORIENTED_EDGE('',*,*,#9497,.T.);
#12875=ORIENTED_EDGE('',*,*,#9503,.T.);
#12876=ORIENTED_EDGE('',*,*,#9504,.F.);
#12877=ORIENTED_EDGE('',*,*,#9505,.T.);
#12878=ORIENTED_EDGE('',*,*,#9501,.T.);
#12879=ORIENTED_EDGE('',*,*,#9506,.T.);
#12880=ORIENTED_EDGE('',*,*,#9507,.F.);
#12881=ORIENTED_EDGE('',*,*,#9508,.T.);
#12882=ORIENTED_EDGE('',*,*,#9504,.T.);
#12883=ORIENTED_EDGE('',*,*,#9509,.T.);
#12884=ORIENTED_EDGE('',*,*,#9510,.F.);
#12885=ORIENTED_EDGE('',*,*,#9511,.T.);
#12886=ORIENTED_EDGE('',*,*,#9507,.T.);
#12887=ORIENTED_EDGE('',*,*,#9512,.T.);
#12888=ORIENTED_EDGE('',*,*,#9513,.F.);
#12889=ORIENTED_EDGE('',*,*,#9514,.T.);
#12890=ORIENTED_EDGE('',*,*,#9510,.T.);
#12891=ORIENTED_EDGE('',*,*,#9515,.T.);
#12892=ORIENTED_EDGE('',*,*,#9516,.F.);
#12893=ORIENTED_EDGE('',*,*,#9517,.T.);
#12894=ORIENTED_EDGE('',*,*,#9513,.T.);
#12895=ORIENTED_EDGE('',*,*,#9518,.T.);
#12896=ORIENTED_EDGE('',*,*,#9519,.F.);
#12897=ORIENTED_EDGE('',*,*,#9520,.T.);
#12898=ORIENTED_EDGE('',*,*,#9516,.T.);
#12899=ORIENTED_EDGE('',*,*,#9521,.T.);
#12900=ORIENTED_EDGE('',*,*,#9522,.F.);
#12901=ORIENTED_EDGE('',*,*,#9523,.T.);
#12902=ORIENTED_EDGE('',*,*,#9519,.T.);
#12903=ORIENTED_EDGE('',*,*,#9524,.T.);
#12904=ORIENTED_EDGE('',*,*,#9525,.F.);
#12905=ORIENTED_EDGE('',*,*,#9526,.T.);
#12906=ORIENTED_EDGE('',*,*,#9522,.T.);
#12907=ORIENTED_EDGE('',*,*,#9527,.T.);
#12908=ORIENTED_EDGE('',*,*,#9528,.F.);
#12909=ORIENTED_EDGE('',*,*,#9529,.T.);
#12910=ORIENTED_EDGE('',*,*,#9525,.T.);
#12911=ORIENTED_EDGE('',*,*,#9530,.T.);
#12912=ORIENTED_EDGE('',*,*,#9531,.F.);
#12913=ORIENTED_EDGE('',*,*,#9532,.T.);
#12914=ORIENTED_EDGE('',*,*,#9528,.T.);
#12915=ORIENTED_EDGE('',*,*,#9533,.T.);
#12916=ORIENTED_EDGE('',*,*,#9534,.F.);
#12917=ORIENTED_EDGE('',*,*,#9535,.T.);
#12918=ORIENTED_EDGE('',*,*,#9536,.F.);
#12919=ORIENTED_EDGE('',*,*,#9537,.F.);
#12920=ORIENTED_EDGE('',*,*,#9538,.F.);
#12921=ORIENTED_EDGE('',*,*,#9539,.T.);
#12922=ORIENTED_EDGE('',*,*,#9534,.T.);
#12923=ORIENTED_EDGE('',*,*,#9540,.F.);
#12924=ORIENTED_EDGE('',*,*,#9541,.F.);
#12925=ORIENTED_EDGE('',*,*,#9542,.T.);
#12926=ORIENTED_EDGE('',*,*,#9538,.T.);
#12927=ORIENTED_EDGE('',*,*,#9543,.F.);
#12928=ORIENTED_EDGE('',*,*,#9544,.F.);
#12929=ORIENTED_EDGE('',*,*,#9545,.T.);
#12930=ORIENTED_EDGE('',*,*,#9541,.T.);
#12931=ORIENTED_EDGE('',*,*,#9546,.F.);
#12932=ORIENTED_EDGE('',*,*,#9547,.F.);
#12933=ORIENTED_EDGE('',*,*,#9548,.T.);
#12934=ORIENTED_EDGE('',*,*,#9544,.T.);
#12935=ORIENTED_EDGE('',*,*,#9549,.F.);
#12936=ORIENTED_EDGE('',*,*,#9550,.F.);
#12937=ORIENTED_EDGE('',*,*,#9551,.T.);
#12938=ORIENTED_EDGE('',*,*,#9547,.T.);
#12939=ORIENTED_EDGE('',*,*,#9552,.F.);
#12940=ORIENTED_EDGE('',*,*,#9553,.F.);
#12941=ORIENTED_EDGE('',*,*,#9554,.T.);
#12942=ORIENTED_EDGE('',*,*,#9550,.T.);
#12943=ORIENTED_EDGE('',*,*,#9555,.F.);
#12944=ORIENTED_EDGE('',*,*,#9556,.F.);
#12945=ORIENTED_EDGE('',*,*,#9557,.T.);
#12946=ORIENTED_EDGE('',*,*,#9553,.T.);
#12947=ORIENTED_EDGE('',*,*,#9558,.F.);
#12948=ORIENTED_EDGE('',*,*,#9559,.F.);
#12949=ORIENTED_EDGE('',*,*,#9560,.T.);
#12950=ORIENTED_EDGE('',*,*,#9556,.T.);
#12951=ORIENTED_EDGE('',*,*,#9561,.F.);
#12952=ORIENTED_EDGE('',*,*,#9562,.F.);
#12953=ORIENTED_EDGE('',*,*,#9563,.T.);
#12954=ORIENTED_EDGE('',*,*,#9559,.T.);
#12955=ORIENTED_EDGE('',*,*,#9564,.F.);
#12956=ORIENTED_EDGE('',*,*,#9565,.F.);
#12957=ORIENTED_EDGE('',*,*,#9566,.T.);
#12958=ORIENTED_EDGE('',*,*,#9562,.T.);
#12959=ORIENTED_EDGE('',*,*,#9567,.F.);
#12960=ORIENTED_EDGE('',*,*,#9568,.T.);
#12961=ORIENTED_EDGE('',*,*,#9569,.T.);
#12962=ORIENTED_EDGE('',*,*,#9570,.T.);
#12963=ORIENTED_EDGE('',*,*,#9571,.T.);
#12964=ORIENTED_EDGE('',*,*,#9569,.F.);
#12965=ORIENTED_EDGE('',*,*,#9570,.F.);
#12966=ORIENTED_EDGE('',*,*,#9571,.F.);
#12967=ORIENTED_EDGE('',*,*,#9572,.T.);
#12968=ORIENTED_EDGE('',*,*,#9573,.F.);
#12969=ORIENTED_EDGE('',*,*,#9574,.F.);
#12970=ORIENTED_EDGE('',*,*,#9572,.F.);
#12971=ORIENTED_EDGE('',*,*,#9568,.F.);
#12972=ORIENTED_EDGE('',*,*,#9575,.T.);
#12973=ORIENTED_EDGE('',*,*,#9576,.T.);
#12974=ORIENTED_EDGE('',*,*,#9577,.T.);
#12975=ORIENTED_EDGE('',*,*,#9499,.F.);
#12976=ORIENTED_EDGE('',*,*,#9573,.T.);
#12977=ORIENTED_EDGE('',*,*,#9574,.T.);
#12978=ORIENTED_EDGE('',*,*,#9578,.T.);
#12979=ORIENTED_EDGE('',*,*,#9579,.T.);
#12980=ORIENTED_EDGE('',*,*,#9580,.T.);
#12981=ORIENTED_EDGE('',*,*,#9578,.F.);
#12982=ORIENTED_EDGE('',*,*,#9579,.F.);
#12983=ORIENTED_EDGE('',*,*,#9580,.F.);
#12984=ORIENTED_EDGE('',*,*,#9581,.T.);
#12985=ORIENTED_EDGE('',*,*,#9582,.T.);
#12986=ORIENTED_EDGE('',*,*,#9581,.F.);
#12987=ORIENTED_EDGE('',*,*,#9536,.T.);
#12988=ORIENTED_EDGE('',*,*,#9583,.T.);
#12989=ORIENTED_EDGE('',*,*,#9584,.F.);
#12990=ORIENTED_EDGE('',*,*,#9585,.F.);
#12991=ORIENTED_EDGE('',*,*,#9586,.T.);
#12992=ORIENTED_EDGE('',*,*,#9586,.F.);
#12993=ORIENTED_EDGE('',*,*,#9587,.F.);
#12994=ORIENTED_EDGE('',*,*,#9533,.F.);
#12995=ORIENTED_EDGE('',*,*,#9530,.F.);
#12996=ORIENTED_EDGE('',*,*,#9527,.F.);
#12997=ORIENTED_EDGE('',*,*,#9524,.F.);
#12998=ORIENTED_EDGE('',*,*,#9521,.F.);
#12999=ORIENTED_EDGE('',*,*,#9518,.F.);
#13000=ORIENTED_EDGE('',*,*,#9515,.F.);
#13001=ORIENTED_EDGE('',*,*,#9512,.F.);
#13002=ORIENTED_EDGE('',*,*,#9509,.F.);
#13003=ORIENTED_EDGE('',*,*,#9506,.F.);
#13004=ORIENTED_EDGE('',*,*,#9503,.F.);
#13005=ORIENTED_EDGE('',*,*,#9500,.F.);
#13006=ORIENTED_EDGE('',*,*,#9577,.F.);
#13007=ORIENTED_EDGE('',*,*,#9588,.T.);
#13008=ORIENTED_EDGE('',*,*,#9567,.T.);
#13009=ORIENTED_EDGE('',*,*,#9564,.T.);
#13010=ORIENTED_EDGE('',*,*,#9561,.T.);
#13011=ORIENTED_EDGE('',*,*,#9558,.T.);
#13012=ORIENTED_EDGE('',*,*,#9555,.T.);
#13013=ORIENTED_EDGE('',*,*,#9552,.T.);
#13014=ORIENTED_EDGE('',*,*,#9549,.T.);
#13015=ORIENTED_EDGE('',*,*,#9546,.T.);
#13016=ORIENTED_EDGE('',*,*,#9543,.T.);
#13017=ORIENTED_EDGE('',*,*,#9540,.T.);
#13018=ORIENTED_EDGE('',*,*,#9537,.T.);
#13019=ORIENTED_EDGE('',*,*,#9565,.T.);
#13020=ORIENTED_EDGE('',*,*,#9588,.F.);
#13021=ORIENTED_EDGE('',*,*,#9576,.F.);
#13022=ORIENTED_EDGE('',*,*,#9589,.T.);
#13023=ORIENTED_EDGE('',*,*,#9583,.F.);
#13024=ORIENTED_EDGE('',*,*,#9535,.F.);
#13025=ORIENTED_EDGE('',*,*,#9539,.F.);
#13026=ORIENTED_EDGE('',*,*,#9542,.F.);
#13027=ORIENTED_EDGE('',*,*,#9545,.F.);
#13028=ORIENTED_EDGE('',*,*,#9548,.F.);
#13029=ORIENTED_EDGE('',*,*,#9551,.F.);
#13030=ORIENTED_EDGE('',*,*,#9554,.F.);
#13031=ORIENTED_EDGE('',*,*,#9557,.F.);
#13032=ORIENTED_EDGE('',*,*,#9560,.F.);
#13033=ORIENTED_EDGE('',*,*,#9563,.F.);
#13034=ORIENTED_EDGE('',*,*,#9566,.F.);
#13035=ORIENTED_EDGE('',*,*,#9589,.F.);
#13036=ORIENTED_EDGE('',*,*,#9575,.F.);
#13037=ORIENTED_EDGE('',*,*,#9498,.F.);
#13038=ORIENTED_EDGE('',*,*,#9502,.F.);
#13039=ORIENTED_EDGE('',*,*,#9505,.F.);
#13040=ORIENTED_EDGE('',*,*,#9508,.F.);
#13041=ORIENTED_EDGE('',*,*,#9511,.F.);
#13042=ORIENTED_EDGE('',*,*,#9514,.F.);
#13043=ORIENTED_EDGE('',*,*,#9517,.F.);
#13044=ORIENTED_EDGE('',*,*,#9520,.F.);
#13045=ORIENTED_EDGE('',*,*,#9523,.F.);
#13046=ORIENTED_EDGE('',*,*,#9526,.F.);
#13047=ORIENTED_EDGE('',*,*,#9529,.F.);
#13048=ORIENTED_EDGE('',*,*,#9532,.F.);
#13049=ORIENTED_EDGE('',*,*,#9590,.F.);
#13050=ORIENTED_EDGE('',*,*,#9531,.T.);
#13051=ORIENTED_EDGE('',*,*,#9587,.T.);
#13052=ORIENTED_EDGE('',*,*,#9591,.F.);
#13053=ORIENTED_EDGE('',*,*,#9590,.T.);
#13054=ORIENTED_EDGE('',*,*,#9592,.T.);
#13055=ORIENTED_EDGE('',*,*,#9593,.T.);
#13056=ORIENTED_EDGE('',*,*,#9594,.F.);
#13057=ORIENTED_EDGE('',*,*,#9593,.F.);
#13058=ORIENTED_EDGE('',*,*,#9595,.F.);
#13059=ORIENTED_EDGE('',*,*,#9594,.T.);
#13060=ORIENTED_EDGE('',*,*,#9582,.F.);
#13061=ORIENTED_EDGE('',*,*,#9596,.T.);
#13062=ORIENTED_EDGE('',*,*,#9595,.T.);
#13063=ORIENTED_EDGE('',*,*,#9596,.F.);
#13064=ORIENTED_EDGE('',*,*,#9597,.F.);
#13065=ORIENTED_EDGE('',*,*,#9598,.T.);
#13066=ORIENTED_EDGE('',*,*,#9584,.T.);
#13067=ORIENTED_EDGE('',*,*,#9591,.T.);
#13068=ORIENTED_EDGE('',*,*,#9585,.T.);
#13069=ORIENTED_EDGE('',*,*,#9598,.F.);
#13070=ORIENTED_EDGE('',*,*,#9597,.T.);
#13071=ORIENTED_EDGE('',*,*,#9599,.F.);
#13072=ORIENTED_EDGE('',*,*,#9599,.T.);
#13073=ORIENTED_EDGE('',*,*,#9600,.T.);
#13074=ORIENTED_EDGE('',*,*,#9601,.F.);
#13075=ORIENTED_EDGE('',*,*,#9600,.F.);
#13076=ORIENTED_EDGE('',*,*,#9602,.F.);
#13077=ORIENTED_EDGE('',*,*,#9601,.T.);
#13078=ORIENTED_EDGE('',*,*,#9602,.T.);
#13079=ORIENTED_EDGE('',*,*,#9603,.T.);
#13080=ORIENTED_EDGE('',*,*,#9604,.F.);
#13081=ORIENTED_EDGE('',*,*,#9603,.F.);
#13082=ORIENTED_EDGE('',*,*,#9604,.T.);
#13083=ORIENTED_EDGE('',*,*,#9592,.F.);
#15502=CONICAL_SURFACE('',#17305,14.9061737618886,1.12276863450922);
#15503=CONICAL_SURFACE('',#17309,19.,0.674740942223553);
#15504=CONICAL_SURFACE('',#17314,22.8438262381114,0.337370471111777);
#15505=CONICAL_SURFACE('',#17330,22.6,0.785398163397437);
#15506=CONICAL_SURFACE('',#17331,11.6,0.785398163397437);
#15964=ADVANCED_FACE('',(#2236),#1689,.T.);
#15965=ADVANCED_FACE('',(#2237),#1690,.T.);
#15966=ADVANCED_FACE('',(#2238),#1691,.T.);
#15967=ADVANCED_FACE('',(#2239),#1692,.T.);
#15968=ADVANCED_FACE('',(#2240),#1693,.T.);
#15969=ADVANCED_FACE('',(#2241),#1694,.T.);
#15970=ADVANCED_FACE('',(#2242),#1695,.T.);
#15971=ADVANCED_FACE('',(#2243),#1696,.T.);
#15972=ADVANCED_FACE('',(#2244),#1697,.T.);
#15973=ADVANCED_FACE('',(#2245),#1698,.T.);
#15974=ADVANCED_FACE('',(#2246),#1699,.T.);
#15975=ADVANCED_FACE('',(#2247),#1700,.T.);
#15976=ADVANCED_FACE('',(#2248),#1701,.T.);
#15977=ADVANCED_FACE('',(#2249),#1702,.T.);
#15978=ADVANCED_FACE('',(#2250),#1703,.T.);
#15979=ADVANCED_FACE('',(#2251),#1704,.T.);
#15980=ADVANCED_FACE('',(#2252),#1705,.T.);
#15981=ADVANCED_FACE('',(#2253),#1706,.T.);
#15982=ADVANCED_FACE('',(#2254),#1707,.T.);
#15983=ADVANCED_FACE('',(#2255),#1708,.T.);
#15984=ADVANCED_FACE('',(#2256),#1709,.T.);
#15985=ADVANCED_FACE('',(#2257),#1710,.T.);
#15986=ADVANCED_FACE('',(#2258),#1711,.T.);
#15987=ADVANCED_FACE('',(#2259),#15502,.T.);
#15988=ADVANCED_FACE('',(#2260),#15503,.T.);
#15989=ADVANCED_FACE('',(#2261,#974),#1219,.T.);
#15990=ADVANCED_FACE('',(#2262),#15504,.T.);
#15991=ADVANCED_FACE('',(#2263),#1712,.T.);
#15992=ADVANCED_FACE('',(#2264),#1220,.F.);
#15993=ADVANCED_FACE('',(#2265),#903,.F.);
#15994=ADVANCED_FACE('',(#2266),#1713,.T.);
#15995=ADVANCED_FACE('',(#2267),#904,.F.);
#15996=ADVANCED_FACE('',(#2268),#1714,.T.);
#15997=ADVANCED_FACE('',(#2269),#1715,.F.);
#15998=ADVANCED_FACE('',(#2270,#975),#1221,.T.);
#15999=ADVANCED_FACE('',(#2271),#15505,.T.);
#16000=ADVANCED_FACE('',(#2272),#15506,.T.);
#16001=ADVANCED_FACE('',(#2273,#976),#1222,.T.);
#16002=ADVANCED_FACE('',(#2274),#1716,.F.);
#16003=ADVANCED_FACE('',(#2275,#977),#1223,.T.);
#16004=ADVANCED_FACE('',(#2276),#1717,.F.);
#16005=ADVANCED_FACE('',(#2277,#978),#1224,.T.);
#16526=CLOSED_SHELL('',(#15964,#15965,#15966,#15967,#15968,#15969,#15970,
#15971,#15972,#15973,#15974,#15975,#15976,#15977,#15978,#15979,#15980,#15981,
#15982,#15983,#15984,#15985,#15986,#15987,#15988,#15989,#15990,#15991,#15992,
#15993,#15994,#15995,#15996,#15997,#15998,#15999,#16000,#16001,#16002,#16003,
#16004,#16005));
#17279=AXIS2_PLACEMENT_3D('',#33388,#19700,#19701);
#17280=AXIS2_PLACEMENT_3D('',#33389,#19702,#19703);
#17281=AXIS2_PLACEMENT_3D('',#33411,#19705,#19706);
#17282=AXIS2_PLACEMENT_3D('',#33422,#19707,#19708);
#17283=AXIS2_PLACEMENT_3D('',#33506,#19710,#19711);
#17284=AXIS2_PLACEMENT_3D('',#33596,#19713,#19714);
#17285=AXIS2_PLACEMENT_3D('',#33686,#19716,#19717);
#17286=AXIS2_PLACEMENT_3D('',#33770,#19719,#19720);
#17287=AXIS2_PLACEMENT_3D('',#33860,#19722,#19723);
#17288=AXIS2_PLACEMENT_3D('',#33950,#19725,#19726);
#17289=AXIS2_PLACEMENT_3D('',#34034,#19728,#19729);
#17290=AXIS2_PLACEMENT_3D('',#34124,#19731,#19732);
#17291=AXIS2_PLACEMENT_3D('',#34214,#19734,#19735);
#17292=AXIS2_PLACEMENT_3D('',#34298,#19737,#19738);
#17293=AXIS2_PLACEMENT_3D('',#34388,#19740,#19741);
#17294=AXIS2_PLACEMENT_3D('',#34409,#19743,#19744);
#17295=AXIS2_PLACEMENT_3D('',#34422,#19745,#19746);
#17296=AXIS2_PLACEMENT_3D('',#34459,#19748,#19749);
#17297=AXIS2_PLACEMENT_3D('',#34496,#19751,#19752);
#17298=AXIS2_PLACEMENT_3D('',#34534,#19754,#19755);
#17299=AXIS2_PLACEMENT_3D('',#34571,#19757,#19758);
#17300=AXIS2_PLACEMENT_3D('',#34608,#19760,#19761);
#17301=AXIS2_PLACEMENT_3D('',#34646,#19763,#19764);
#17302=AXIS2_PLACEMENT_3D('',#34683,#19766,#19767);
#17303=AXIS2_PLACEMENT_3D('',#34720,#19769,#19770);
#17304=AXIS2_PLACEMENT_3D('',#34758,#19772,#19773);
#17305=AXIS2_PLACEMENT_3D('',#34795,#19775,#19776);
#17306=AXIS2_PLACEMENT_3D('',#34797,#19777,#19778);
#17307=AXIS2_PLACEMENT_3D('',#34801,#19780,#19781);
#17308=AXIS2_PLACEMENT_3D('',#34802,#19782,#19783);
#17309=AXIS2_PLACEMENT_3D('',#34803,#19784,#19785);
#17310=AXIS2_PLACEMENT_3D('',#34807,#19787,#19788);
#17311=AXIS2_PLACEMENT_3D('',#34808,#19789,#19790);
#17312=AXIS2_PLACEMENT_3D('',#34809,#19791,#19792);
#17313=AXIS2_PLACEMENT_3D('',#34942,#19793,#19794);
#17314=AXIS2_PLACEMENT_3D('',#35073,#19795,#19796);
#17315=AXIS2_PLACEMENT_3D('',#35077,#19798,#19799);
#17316=AXIS2_PLACEMENT_3D('',#35078,#19800,#19801);
#17317=AXIS2_PLACEMENT_3D('',#35079,#19802,#19803);
#17318=AXIS2_PLACEMENT_3D('',#35082,#19805,#19806);
#17319=AXIS2_PLACEMENT_3D('',#35083,#19807,#19808);
#17320=AXIS2_PLACEMENT_3D('',#35216,#19809,#19810);
#17321=AXIS2_PLACEMENT_3D('',#35218,#19811,#19812);
#17322=AXIS2_PLACEMENT_3D('',#35991,#19813,#19814);
#17323=AXIS2_PLACEMENT_3D('',#36626,#19815,#19816);
#17324=AXIS2_PLACEMENT_3D('',#36627,#19817,#19818);
#17325=AXIS2_PLACEMENT_3D('',#36628,#19819,#19820);
#17326=AXIS2_PLACEMENT_3D('',#36630,#19821,#19822);
#17327=AXIS2_PLACEMENT_3D('',#36633,#19824,#19825);
#17328=AXIS2_PLACEMENT_3D('',#36634,#19826,#19827);
#17329=AXIS2_PLACEMENT_3D('',#36636,#19828,#19829);
#17330=AXIS2_PLACEMENT_3D('',#36637,#19830,#19831);
#17331=AXIS2_PLACEMENT_3D('',#36639,#19833,#19834);
#17332=AXIS2_PLACEMENT_3D('',#36641,#19835,#19836);
#17333=AXIS2_PLACEMENT_3D('',#36643,#19838,#19839);
#17334=AXIS2_PLACEMENT_3D('',#36645,#19840,#19841);
#17335=AXIS2_PLACEMENT_3D('',#36646,#19842,#19843);
#17336=AXIS2_PLACEMENT_3D('',#36649,#19845,#19846);
#17337=AXIS2_PLACEMENT_3D('',#36650,#19847,#19848);
#17338=AXIS2_PLACEMENT_3D('',#36652,#19849,#19850);
#17339=AXIS2_PLACEMENT_3D('',#36653,#19851,#19852);
#17340=AXIS2_PLACEMENT_3D('',#36656,#19854,#19855);
#17341=AXIS2_PLACEMENT_3D('',#36657,#19856,#19857);
#19700=DIRECTION('axis',(0.,0.,1.));
#19701=DIRECTION('refdir',(1.,0.,0.));
#19702=DIRECTION('center_axis',(1.,0.,0.));
#19703=DIRECTION('ref_axis',(0.,1.,0.));
#19704=DIRECTION('',(-1.,0.,0.));
#19705=DIRECTION('center_axis',(-1.,0.,0.));
#19706=DIRECTION('ref_axis',(0.,1.,0.));
#19707=DIRECTION('center_axis',(1.,0.,0.));
#19708=DIRECTION('ref_axis',(0.,1.,0.));
#19709=DIRECTION('',(-1.,0.,0.));
#19710=DIRECTION('center_axis',(1.,0.,0.));
#19711=DIRECTION('ref_axis',(0.,1.,0.));
#19712=DIRECTION('',(-1.,0.,0.));
#19713=DIRECTION('center_axis',(1.,0.,0.));
#19714=DIRECTION('ref_axis',(0.,1.,0.));
#19715=DIRECTION('',(-1.,0.,0.));
#19716=DIRECTION('center_axis',(1.,0.,0.));
#19717=DIRECTION('ref_axis',(0.,1.,0.));
#19718=DIRECTION('',(-1.,0.,0.));
#19719=DIRECTION('center_axis',(1.,0.,0.));
#19720=DIRECTION('ref_axis',(0.,1.,0.));
#19721=DIRECTION('',(-1.,0.,0.));
#19722=DIRECTION('center_axis',(1.,0.,0.));
#19723=DIRECTION('ref_axis',(0.,1.,0.));
#19724=DIRECTION('',(-1.,0.,0.));
#19725=DIRECTION('center_axis',(1.,0.,0.));
#19726=DIRECTION('ref_axis',(0.,1.,0.));
#19727=DIRECTION('',(-1.,0.,0.));
#19728=DIRECTION('center_axis',(1.,0.,0.));
#19729=DIRECTION('ref_axis',(0.,1.,0.));
#19730=DIRECTION('',(-1.,0.,0.));
#19731=DIRECTION('center_axis',(1.,0.,0.));
#19732=DIRECTION('ref_axis',(0.,1.,0.));
#19733=DIRECTION('',(-1.,0.,0.));
#19734=DIRECTION('center_axis',(1.,0.,0.));
#19735=DIRECTION('ref_axis',(0.,1.,0.));
#19736=DIRECTION('',(-1.,0.,0.));
#19737=DIRECTION('center_axis',(1.,0.,0.));
#19738=DIRECTION('ref_axis',(0.,1.,0.));
#19739=DIRECTION('',(-1.,0.,0.));
#19740=DIRECTION('center_axis',(1.,0.,0.));
#19741=DIRECTION('ref_axis',(0.,1.,5.00345854329736E-14));
#19742=DIRECTION('',(1.,0.,0.));
#19743=DIRECTION('center_axis',(1.,0.,0.));
#19744=DIRECTION('ref_axis',(0.,1.,5.00345854329736E-14));
#19745=DIRECTION('center_axis',(1.,0.,0.));
#19746=DIRECTION('ref_axis',(0.,1.,5.00345854329736E-14));
#19747=DIRECTION('',(1.,0.,0.));
#19748=DIRECTION('center_axis',(1.,0.,0.));
#19749=DIRECTION('ref_axis',(0.,1.,5.00345854329736E-14));
#19750=DIRECTION('',(1.,0.,0.));
#19751=DIRECTION('center_axis',(1.,0.,0.));
#19752=DIRECTION('ref_axis',(0.,1.,5.00345854329736E-14));
#19753=DIRECTION('',(1.,0.,0.));
#19754=DIRECTION('center_axis',(1.,0.,0.));
#19755=DIRECTION('ref_axis',(0.,1.,5.00345854329736E-14));
#19756=DIRECTION('',(1.,0.,0.));
#19757=DIRECTION('center_axis',(1.,0.,0.));
#19758=DIRECTION('ref_axis',(0.,1.,5.00345854329736E-14));
#19759=DIRECTION('',(1.,0.,0.));
#19760=DIRECTION('center_axis',(1.,0.,0.));
#19761=DIRECTION('ref_axis',(0.,1.,5.00345854329736E-14));
#19762=DIRECTION('',(1.,0.,0.));
#19763=DIRECTION('center_axis',(1.,0.,0.));
#19764=DIRECTION('ref_axis',(0.,1.,5.00345854329736E-14));
#19765=DIRECTION('',(1.,0.,0.));
#19766=DIRECTION('center_axis',(1.,0.,0.));
#19767=DIRECTION('ref_axis',(0.,1.,5.00345854329736E-14));
#19768=DIRECTION('',(1.,0.,0.));
#19769=DIRECTION('center_axis',(1.,0.,0.));
#19770=DIRECTION('ref_axis',(0.,1.,5.00345854329736E-14));
#19771=DIRECTION('',(1.,0.,0.));
#19772=DIRECTION('center_axis',(1.,0.,0.));
#19773=DIRECTION('ref_axis',(0.,1.,5.00345854329736E-14));
#19774=DIRECTION('',(1.,0.,0.));
#19775=DIRECTION('center_axis',(-1.,0.,-2.40145555254033E-15));
#19776=DIRECTION('ref_axis',(0.,-1.,-3.14504206142599E-17));
#19777=DIRECTION('center_axis',(-1.,0.,0.));
#19778=DIRECTION('ref_axis',(0.,-1.,0.));
#19779=DIRECTION('',(-0.433188730489141,0.901303236306853,-9.01559303907765E-16));
#19780=DIRECTION('center_axis',(1.,0.,0.));
#19781=DIRECTION('ref_axis',(0.,-1.,-6.12323399573677E-17));
#19782=DIRECTION('center_axis',(1.,0.,0.));
#19783=DIRECTION('ref_axis',(0.,-1.,-6.12323399573677E-17));
#19784=DIRECTION('center_axis',(-1.,0.,0.));
#19785=DIRECTION('ref_axis',(0.,1.,0.));
#19786=DIRECTION('',(-0.78086880944303,-0.624695047554424,-7.65030790430729E-17));
#19787=DIRECTION('center_axis',(-1.,0.,0.));
#19788=DIRECTION('ref_axis',(0.,-1.,-6.12323399573677E-17));
#19789=DIRECTION('center_axis',(-1.,0.,0.));
#19790=DIRECTION('ref_axis',(0.,-1.,-6.12323399573677E-17));
#19791=DIRECTION('center_axis',(1.,0.,0.));
#19792=DIRECTION('ref_axis',(0.,0.,-1.));
#19793=DIRECTION('center_axis',(-1.,0.,0.));
#19794=DIRECTION('ref_axis',(0.,1.,5.00345854329736E-14));
#19795=DIRECTION('center_axis',(-1.,0.,1.56015765102107E-15));
#19796=DIRECTION('ref_axis',(0.,-1.,-3.04068599274537E-17));
#19797=DIRECTION('',(-0.943628319160417,0.331006941435501,1.52281048269397E-15));
#19798=DIRECTION('center_axis',(1.,0.,0.));
#19799=DIRECTION('ref_axis',(0.,-1.,0.));
#19800=DIRECTION('center_axis',(1.,0.,0.));
#19801=DIRECTION('ref_axis',(0.,-1.,0.));
#19802=DIRECTION('center_axis',(1.,0.,0.));
#19803=DIRECTION('ref_axis',(0.,1.,0.));
#19804=DIRECTION('',(-1.,0.,0.));
#19805=DIRECTION('center_axis',(1.,0.,0.));
#19806=DIRECTION('ref_axis',(0.,0.,-1.));
#19807=DIRECTION('center_axis',(1.,0.,0.));
#19808=DIRECTION('ref_axis',(0.,0.,-1.));
#19809=DIRECTION('center_axis',(-1.,0.,0.));
#19810=DIRECTION('ref_axis',(0.,1.,0.));
#19811=DIRECTION('center_axis',(-1.,0.,0.));
#19812=DIRECTION('ref_axis',(0.,1.,0.));
#19813=DIRECTION('center_axis',(1.,0.,0.));
#19814=DIRECTION('ref_axis',(0.,0.888975527931182,0.457954703807566));
#19815=DIRECTION('center_axis',(1.,0.,0.));
#19816=DIRECTION('ref_axis',(0.,-0.48878186078128,-0.872406036528398));
#19817=DIRECTION('center_axis',(-1.,0.,0.));
#19818=DIRECTION('ref_axis',(0.,1.,0.));
#19819=DIRECTION('center_axis',(1.,0.,0.));
#19820=DIRECTION('ref_axis',(0.,1.,0.));
#19821=DIRECTION('center_axis',(1.,0.,0.));
#19822=DIRECTION('ref_axis',(0.,0.,-1.));
#19823=DIRECTION('',(-1.,0.,0.));
#19824=DIRECTION('center_axis',(1.,0.,0.));
#19825=DIRECTION('ref_axis',(0.,0.,-1.));
#19826=DIRECTION('center_axis',(-1.,0.,0.));
#19827=DIRECTION('ref_axis',(0.,0.,1.));
#19828=DIRECTION('center_axis',(1.,0.,0.));
#19829=DIRECTION('ref_axis',(0.,0.,-1.));
#19830=DIRECTION('center_axis',(1.,0.,0.));
#19831=DIRECTION('ref_axis',(0.,1.,0.));
#19832=DIRECTION('',(-0.707106781186555,0.70710678118654,8.65956056235484E-17));
#19833=DIRECTION('center_axis',(-1.,0.,0.));
#19834=DIRECTION('ref_axis',(0.,1.,0.));
#19835=DIRECTION('center_axis',(1.,0.,0.));
#19836=DIRECTION('ref_axis',(0.,0.,-1.));
#19837=DIRECTION('',(-0.707106781186555,-0.70710678118654,-8.65956056235484E-17));
#19838=DIRECTION('center_axis',(1.,0.,0.));
#19839=DIRECTION('ref_axis',(0.,0.,-1.));
#19840=DIRECTION('center_axis',(1.,0.,0.));
#19841=DIRECTION('ref_axis',(0.,0.,-1.));
#19842=DIRECTION('center_axis',(1.,0.,0.));
#19843=DIRECTION('ref_axis',(0.,1.,0.));
#19844=DIRECTION('',(-1.,0.,0.));
#19845=DIRECTION('center_axis',(1.,0.,0.));
#19846=DIRECTION('ref_axis',(0.,0.,-1.));
#19847=DIRECTION('center_axis',(-1.,0.,0.));
#19848=DIRECTION('ref_axis',(0.,0.,1.));
#19849=DIRECTION('center_axis',(1.,0.,0.));
#19850=DIRECTION('ref_axis',(0.,0.,-1.));
#19851=DIRECTION('center_axis',(1.,0.,0.));
#19852=DIRECTION('ref_axis',(0.,1.,0.));
#19853=DIRECTION('',(-1.,0.,0.));
#19854=DIRECTION('center_axis',(1.,0.,0.));
#19855=DIRECTION('ref_axis',(0.,0.,-1.));
#19856=DIRECTION('center_axis',(1.,0.,0.));
#19857=DIRECTION('ref_axis',(0.,0.,-1.));
#33388=CARTESIAN_POINT('',(0.,0.,0.));
#33389=CARTESIAN_POINT('Origin',(212.6,0.,0.));
#33390=CARTESIAN_POINT('',(204.481156847152,-11.9249052711737,0.000302535951811622));
#33391=CARTESIAN_POINT('',(204.268843152848,-11.9248035800407,0.000218476360169007));
#33392=CARTESIAN_POINT('',(212.6,-11.925,-1.46039130798322E-15));
#33393=CARTESIAN_POINT('',(204.,5.12964461189265,10.7653319110783));
#33394=CARTESIAN_POINT('Ctrl Pts',(204.481156847152,-11.9249052711737,0.000302535951811622));
#33395=CARTESIAN_POINT('Ctrl Pts',(204.471375386274,-11.9253914263212,0.488902467455807));
#33396=CARTESIAN_POINT('Ctrl Pts',(204.461593925397,-11.8959222415045,0.977444055122396));
#33397=CARTESIAN_POINT('Ctrl Pts',(204.451812464519,-11.8360320098832,1.46222727880249));
#33398=CARTESIAN_POINT('Ctrl Pts',(204.412321413966,-11.5942349824066,3.41946035810522));
#33399=CARTESIAN_POINT('Ctrl Pts',(204.372830363414,-10.8565722369881,5.31543177641324));
#33400=CARTESIAN_POINT('Ctrl Pts',(204.333339312861,-9.71202673712791,6.92143673402461));
#33401=CARTESIAN_POINT('Ctrl Pts',(204.293848262308,-8.56748123726774,8.52744169163597));
#33402=CARTESIAN_POINT('Ctrl Pts',(204.254357211755,-7.01605298296593,9.84348018855067));
#33403=CARTESIAN_POINT('Ctrl Pts',(204.214866161202,-5.24489388990008,10.7107847596565));
#33404=CARTESIAN_POINT('Ctrl Pts',(204.17537511065,-3.47373479683424,11.5780893307624));
#33405=CARTESIAN_POINT('Ctrl Pts',(204.135884060097,-1.48284486500436,11.9966599760593));
#33406=CARTESIAN_POINT('Ctrl Pts',(204.096393009544,0.487620662860904,11.9160328022271));
#33407=CARTESIAN_POINT('Ctrl Pts',(204.064262006363,2.09084552668397,11.850432319519));
#33408=CARTESIAN_POINT('Ctrl Pts',(204.032131003181,3.68054964658133,11.4543680498425));
#33409=CARTESIAN_POINT('Ctrl Pts',(204.,5.1300262208937,10.7654810839693));
#33410=CARTESIAN_POINT('',(204.,-5.12964461189138,10.7653319110789));
#33411=CARTESIAN_POINT('Origin',(204.,0.,0.));
#33412=CARTESIAN_POINT('Ctrl Pts',(204.,-5.12964461189138,10.7653319110789));
#33413=CARTESIAN_POINT('Ctrl Pts',(204.039491050553,-6.91044286403787,9.91678750627631));
#33414=CARTESIAN_POINT('Ctrl Pts',(204.078982101106,-8.47572680110246,8.61820334451372));
#33415=CARTESIAN_POINT('Ctrl Pts',(204.118473151658,-9.63736634999488,7.02480970362073));
#33416=CARTESIAN_POINT('Ctrl Pts',(204.157964202211,-10.7990058988873,5.43141606272772));
#33417=CARTESIAN_POINT('Ctrl Pts',(204.197455252764,-11.5570010596076,3.54321294270431));
#33418=CARTESIAN_POINT('Ctrl Pts',(204.236946303317,-11.8197391311641,1.58862178928765));
#33419=CARTESIAN_POINT('Ctrl Pts',(204.247578586494,-11.8904768182884,1.06238188561764));
#33420=CARTESIAN_POINT('Ctrl Pts',(204.258210869671,-11.9253151710161,0.531329761662712));
#33421=CARTESIAN_POINT('Ctrl Pts',(204.268843152848,-11.9248035800407,0.000218476360169007));
#33422=CARTESIAN_POINT('Origin',(212.6,0.,0.));
#33423=CARTESIAN_POINT('',(205.981156847152,-11.9257948710858,-0.00017386328305502));
#33424=CARTESIAN_POINT('',(205.768843152848,-11.925879493633,-0.000136868446097685));
#33425=CARTESIAN_POINT('',(212.6,-11.925,-1.46039130798322E-15));
#33426=CARTESIAN_POINT('Ctrl Pts',(205.981156847152,-11.9257948710858,-0.00017386328305502));
#33427=CARTESIAN_POINT('Ctrl Pts',(205.945267992908,-11.9245188658506,1.79214687948621));
#33428=CARTESIAN_POINT('Ctrl Pts',(205.909379138663,-11.5147464964249,3.58503144351514));
#33429=CARTESIAN_POINT('Ctrl Pts',(205.873490284419,-10.7335884774596,5.19806139375664));
#33430=CARTESIAN_POINT('Ctrl Pts',(205.833999233866,-9.87402493144417,6.97299259870679));
#33431=CARTESIAN_POINT('Ctrl Pts',(205.794508183313,-8.56478166178296,8.53015294168481));
#33432=CARTESIAN_POINT('Ctrl Pts',(205.755017132761,-6.96379286278294,9.68170195869235));
#33433=CARTESIAN_POINT('Ctrl Pts',(205.715526082208,-5.36280406378292,10.8332509756999));
#33434=CARTESIAN_POINT('Ctrl Pts',(205.676035031655,-3.47006973544408,11.579188666737));
#33435=CARTESIAN_POINT('Ctrl Pts',(205.636543981102,-1.51391067883033,11.8295324642507));
#33436=CARTESIAN_POINT('Ctrl Pts',(205.59705293055,0.442248377783413,12.0798762617644));
#33437=CARTESIAN_POINT('Ctrl Pts',(205.557561879997,2.46183216267207,11.8346261657547));
#33438=CARTESIAN_POINT('Ctrl Pts',(205.518070829444,4.30121800879738,11.1233667329109));
#33439=CARTESIAN_POINT('Ctrl Pts',(205.478579778891,6.14060385492269,10.4121073000672));
#33440=CARTESIAN_POINT('Ctrl Pts',(205.439088728338,7.79979176228466,9.23483853038924));
#33441=CARTESIAN_POINT('Ctrl Pts',(205.399597677786,9.07863366507509,7.73357450785956));
#33442=CARTESIAN_POINT('Ctrl Pts',(205.360106627233,10.3574755678655,6.23231048532987));
#33443=CARTESIAN_POINT('Ctrl Pts',(205.32061557668,11.2559714660844,4.40705120994843));
#33444=CARTESIAN_POINT('Ctrl Pts',(205.281124526127,11.6657356806046,2.47797797538542));
#33445=CARTESIAN_POINT('Ctrl Pts',(205.241633475575,12.0754998951248,0.548904740822421));
#33446=CARTESIAN_POINT('Ctrl Pts',(205.202142425022,11.9965324259463,-1.48398245292214));
#33447=CARTESIAN_POINT('Ctrl Pts',(205.162651374469,11.43835912164,-3.37545618326797));
#33448=CARTESIAN_POINT('Ctrl Pts',(205.123160323916,10.8801858173337,-5.2669299136138));
#33449=CARTESIAN_POINT('Ctrl Pts',(205.083669273363,9.84280667789951,-7.01699018056091));
#33450=CARTESIAN_POINT('Ctrl Pts',(205.044178222811,8.45136090743825,-8.41452689692128));
#33451=CARTESIAN_POINT('Ctrl Pts',(205.004687172258,7.059915136977,-9.81206361328165));
#33452=CARTESIAN_POINT('Ctrl Pts',(204.965196121705,5.31440273548863,-10.8570767790553));
#33453=CARTESIAN_POINT('Ctrl Pts',(204.925705071152,3.42538506743283,-11.4235064763634));
#33454=CARTESIAN_POINT('Ctrl Pts',(204.8862140206,1.53636739937703,-11.9899361736716));
#33455=CARTESIAN_POINT('Ctrl Pts',(204.846722970047,-0.496155535246199,
-12.0777824025142));
#33456=CARTESIAN_POINT('Ctrl Pts',(204.807231919494,-2.42700014393072,-11.6764479195652));
#33457=CARTESIAN_POINT('Ctrl Pts',(204.767740868941,-4.35784475261525,-11.2751134366161));
#33458=CARTESIAN_POINT('Ctrl Pts',(204.728249818389,-6.18701103536108,-10.3845982418754));
#33459=CARTESIAN_POINT('Ctrl Pts',(204.688758767836,-7.69384656645438,-9.11232601683176));
#33460=CARTESIAN_POINT('Ctrl Pts',(204.649267717283,-9.20068209754767,-7.84005379178813));
#33461=CARTESIAN_POINT('Ctrl Pts',(204.60977666673,-10.3851868769884,-6.18602453644161));
#33462=CARTESIAN_POINT('Ctrl Pts',(204.570285616177,-11.1044736119415,-4.34976253861964));
#33463=CARTESIAN_POINT('Ctrl Pts',(204.540576026502,-11.6456016258877,-2.96832067450525));
#33464=CARTESIAN_POINT('Ctrl Pts',(204.510866436827,-11.9234286543235,-1.48373994625058));
#33465=CARTESIAN_POINT('Ctrl Pts',(204.481156847152,-11.9249052711737,0.000302535951811622));
#33466=CARTESIAN_POINT('Ctrl Pts',(204.268843152848,-11.9248035800407,0.000218476360169007));
#33467=CARTESIAN_POINT('Ctrl Pts',(204.297701920224,-11.9234149897725,-1.44135496348323));
#33468=CARTESIAN_POINT('Ctrl Pts',(204.326560687599,-11.6615962792732,-2.88336425683184));
#33469=CARTESIAN_POINT('Ctrl Pts',(204.355419454975,-11.1503333329718,-4.23076491755909));
#33470=CARTESIAN_POINT('Ctrl Pts',(204.394910505528,-10.4507084808302,-6.07458128417927));
#33471=CARTESIAN_POINT('Ctrl Pts',(204.43440155608,-9.28397779415416,-7.7412348306097));
#33472=CARTESIAN_POINT('Ctrl Pts',(204.473892606633,-7.7908367643509,-9.02955893682934));
#33473=CARTESIAN_POINT('Ctrl Pts',(204.513383657186,-6.29769573454765,-10.317883043049));
#33474=CARTESIAN_POINT('Ctrl Pts',(204.552874707739,-4.47814436161721,-11.2278777090578));
#33475=CARTESIAN_POINT('Ctrl Pts',(204.592365758292,-2.55169822806604,-11.6498261182712));
#33476=CARTESIAN_POINT('Ctrl Pts',(204.631856808844,-0.625252094514863,
-12.0717745274846));
#33477=CARTESIAN_POINT('Ctrl Pts',(204.671347859397,1.40808879965704,-12.0056766799026));
#33478=CARTESIAN_POINT('Ctrl Pts',(204.71083890995,3.30305318516678,-11.4594791445967));
#33479=CARTESIAN_POINT('Ctrl Pts',(204.750329960503,5.19801757067652,-10.9132816092908));
#33480=CARTESIAN_POINT('Ctrl Pts',(204.789821011055,6.9546054475241,-9.886984386261));
#33481=CARTESIAN_POINT('Ctrl Pts',(204.829312061608,8.36091415185001,-8.50440268311452));
#33482=CARTESIAN_POINT('Ctrl Pts',(204.868803112161,9.76722285617592,-7.12182097996805));
#33483=CARTESIAN_POINT('Ctrl Pts',(204.908294162714,10.8232523879802,-5.38295479670486));
#33484=CARTESIAN_POINT('Ctrl Pts',(204.947785213267,11.401616262652,-3.49755765611992));
#33485=CARTESIAN_POINT('Ctrl Pts',(204.987276263819,11.9799801373238,-1.61216051553499));
#33486=CARTESIAN_POINT('Ctrl Pts',(205.026767314372,12.0806783548632,0.419767582371721));
#33487=CARTESIAN_POINT('Ctrl Pts',(205.066258364925,11.6915624780006,2.3531119337468));
#33488=CARTESIAN_POINT('Ctrl Pts',(205.105749415478,11.3024466011381,4.28645628512189));
#33489=CARTESIAN_POINT('Ctrl Pts',(205.14524046603,10.4235166298735,6.12121688996534));
#33490=CARTESIAN_POINT('Ctrl Pts',(205.184731516583,9.16079857987295,7.63606773280669));
#33491=CARTESIAN_POINT('Ctrl Pts',(205.224222567136,7.89808052987239,9.15091857564802));
#33492=CARTESIAN_POINT('Ctrl Pts',(205.263713617689,6.25157440113582,10.3458596564872));
#33493=CARTESIAN_POINT('Ctrl Pts',(205.303204668241,4.41989817863815,11.0767443960842));
#33494=CARTESIAN_POINT('Ctrl Pts',(205.342695718794,2.58822195614046,11.8076291356812));
#33495=CARTESIAN_POINT('Ctrl Pts',(205.382186769347,0.571375639881673,12.0744575340359));
#33496=CARTESIAN_POINT('Ctrl Pts',(205.4216778199,-1.38734819215102,11.8450423672815));
#33497=CARTESIAN_POINT('Ctrl Pts',(205.461168870453,-3.34607202418372,11.615627200527));
#33498=CARTESIAN_POINT('Ctrl Pts',(205.500659921005,-5.24667337199031,10.8899684686634));
#33499=CARTESIAN_POINT('Ctrl Pts',(205.540150971558,-6.85988249812762,9.75560232941972));
#33500=CARTESIAN_POINT('Ctrl Pts',(205.579642022111,-8.47309162426492,8.62123619017606));
#33501=CARTESIAN_POINT('Ctrl Pts',(205.619133072664,-9.79890852873291,7.07816264355239));
#33502=CARTESIAN_POINT('Ctrl Pts',(205.658624123216,-10.6773997071198,5.31252293613964));
#33503=CARTESIAN_POINT('Ctrl Pts',(205.69536379976,-11.4946856817605,3.66989680096673));
#33504=CARTESIAN_POINT('Ctrl Pts',(205.732103476304,-11.9248057040004,1.83463689896584));
#33505=CARTESIAN_POINT('Ctrl Pts',(205.768843152848,-11.925879493633,-0.000136868446097685));
#33506=CARTESIAN_POINT('Origin',(212.6,0.,0.));
#33507=CARTESIAN_POINT('',(207.481156847152,-11.9240882605208,-0.000122447896127587));
#33508=CARTESIAN_POINT('',(207.268843152848,-11.9241429677904,-0.000156968565329557));
#33509=CARTESIAN_POINT('',(212.6,-11.925,-1.46039130798322E-15));
#33510=CARTESIAN_POINT('Ctrl Pts',(207.481156847152,-11.9240882605208,-0.000122447896127587));
#33511=CARTESIAN_POINT('Ctrl Pts',(207.458651650094,-11.9236789998492,1.12426988415646));
#33512=CARTESIAN_POINT('Ctrl Pts',(207.436146453035,-11.7658768963148,2.24877473613482));
#33513=CARTESIAN_POINT('Ctrl Pts',(207.413641255977,-11.4522567635277,3.32799923052405));
#33514=CARTESIAN_POINT('Ctrl Pts',(207.374150205424,-10.9019310549283,5.22177109821098));
#33515=CARTESIAN_POINT('Ctrl Pts',(207.334659154872,-9.87181728028402,6.97611766767221));
#33516=CARTESIAN_POINT('Ctrl Pts',(207.295168104319,-8.48617820498044,8.37941187252719));
#33517=CARTESIAN_POINT('Ctrl Pts',(207.255677053766,-7.10053912967688,9.78270607738215));
#33518=CARTESIAN_POINT('Ctrl Pts',(207.216186003213,-5.35937475371405,10.8349479176309));
#33519=CARTESIAN_POINT('Ctrl Pts',(207.17669495266,-3.47272197366958,11.4092053163104));
#33520=CARTESIAN_POINT('Ctrl Pts',(207.137203902108,-1.5860691936251,11.98346271499));
#33521=CARTESIAN_POINT('Ctrl Pts',(207.097712851555,0.446071990500981,12.0797356721004));
#33522=CARTESIAN_POINT('Ctrl Pts',(207.058221801002,2.3785641100045,11.6864107676709));
#33523=CARTESIAN_POINT('Ctrl Pts',(207.018730750449,4.31105622950802,11.2930858632414));
#33524=CARTESIAN_POINT('Ctrl Pts',(206.979239699897,6.14389928438897,10.4101630972718));
#33525=CARTESIAN_POINT('Ctrl Pts',(206.939748649344,7.65599716650529,9.14414956366061));
#33526=CARTESIAN_POINT('Ctrl Pts',(206.900257598791,9.16809504862161,7.87813603004939));
#33527=CARTESIAN_POINT('Ctrl Pts',(206.860766548238,10.3594477579733,6.22903172879648));
#33528=CARTESIAN_POINT('Ctrl Pts',(206.821275497686,11.0863422544498,4.39576833708731));
#33529=CARTESIAN_POINT('Ctrl Pts',(206.781784447133,11.8132367509262,2.56250494537814));
#33530=CARTESIAN_POINT('Ctrl Pts',(206.74229339658,12.0756730345274,0.545082463212723));
#33531=CARTESIAN_POINT('Ctrl Pts',(206.702802346027,11.8419933805049,-1.41313715973078));
#33532=CARTESIAN_POINT('Ctrl Pts',(206.663311295474,11.6083137264823,-3.37135678267428));
#33533=CARTESIAN_POINT('Ctrl Pts',(206.623820244922,10.8785181348361,-5.27037354639587));
#33534=CARTESIAN_POINT('Ctrl Pts',(206.584329194369,9.74064194750141,-6.8811087992197));
#33535=CARTESIAN_POINT('Ctrl Pts',(206.544838143816,8.60276576016673,-8.49184405204354));
#33536=CARTESIAN_POINT('Ctrl Pts',(206.505347093263,7.05680897714361,-9.8142977939696));
#33537=CARTESIAN_POINT('Ctrl Pts',(206.465856042711,5.28926057640347,-10.6889422494037));
#33538=CARTESIAN_POINT('Ctrl Pts',(206.426364992158,3.52171217566333,-11.5635867048377));
#33539=CARTESIAN_POINT('Ctrl Pts',(206.386873941605,1.53257215720617,-11.9904218737798));
#33540=CARTESIAN_POINT('Ctrl Pts',(206.347382891052,-0.438209246759027,
-11.917958571503));
#33541=CARTESIAN_POINT('Ctrl Pts',(206.307891840499,-2.40899065072422,-11.8454952692263));
#33542=CARTESIAN_POINT('Ctrl Pts',(206.268400789947,-4.36141344019744,-11.2737334957307));
#33543=CARTESIAN_POINT('Ctrl Pts',(206.228909739394,-6.05995658730328,-10.2716449518268));
#33544=CARTESIAN_POINT('Ctrl Pts',(206.189418688841,-7.75849973440911,-9.26955640792297));
#33545=CARTESIAN_POINT('Ctrl Pts',(206.149927638288,-9.20316323914755,-7.83714109361087));
#33546=CARTESIAN_POINT('Ctrl Pts',(206.110436587736,-10.2196771455715,-6.14719146407803));
#33547=CARTESIAN_POINT('Ctrl Pts',(206.070945537183,-11.2361910519954,-4.45724183454519));
#33548=CARTESIAN_POINT('Ctrl Pts',(206.03145448663,-11.8245553601048,-2.50975788979161));
#33549=CARTESIAN_POINT('Ctrl Pts',(205.991963436077,-11.9137956029747,-0.539664883953685));
#33550=CARTESIAN_POINT('Ctrl Pts',(205.988361239769,-11.9219356972222,-0.359961846084769));
#33551=CARTESIAN_POINT('Ctrl Pts',(205.98475904346,-11.9259229448693,-0.180070694740662));
#33552=CARTESIAN_POINT('Ctrl Pts',(205.981156847152,-11.9257948710858,-0.00017386328305502));
#33553=CARTESIAN_POINT('Ctrl Pts',(205.768843152848,-11.925879493633,-0.000136868446097685));
#33554=CARTESIAN_POINT('Ctrl Pts',(205.771594526857,-11.9259599079742,-0.137540061143698));
#33555=CARTESIAN_POINT('Ctrl Pts',(205.774345900866,-11.923634116918,-0.274940527469211));
#33556=CARTESIAN_POINT('Ctrl Pts',(205.777097274875,-11.9188845310052,-0.412257158256467));
#33557=CARTESIAN_POINT('Ctrl Pts',(205.816588325427,-11.8507127241981,-2.38319167703802));
#33558=CARTESIAN_POINT('Ctrl Pts',(205.85607937598,-11.2832036582781,-4.33685484639931));
#33559=CARTESIAN_POINT('Ctrl Pts',(205.895570426533,-10.2848160225208,-6.03757599437023));
#33560=CARTESIAN_POINT('Ctrl Pts',(205.935061477086,-9.28642838676358,-7.73829714234115));
#33561=CARTESIAN_POINT('Ctrl Pts',(205.974552527639,-7.85716218116911,-9.18607626892171));
#33562=CARTESIAN_POINT('Ctrl Pts',(206.014043578191,-6.16942998670385,-10.2062675883473));
#33563=CARTESIAN_POINT('Ctrl Pts',(206.053534628744,-4.48169779223858,-11.2264589077728));
#33564=CARTESIAN_POINT('Ctrl Pts',(206.093025679297,-2.53549960890252,-11.8190624200434));
#33565=CARTESIAN_POINT('Ctrl Pts',(206.13251672985,-0.565605587893831,-11.9125922786295));
#33566=CARTESIAN_POINT('Ctrl Pts',(206.172007780402,1.40428843311484,-12.0061221372157));
#33567=CARTESIAN_POINT('Ctrl Pts',(206.211498830955,3.39787829179614,-11.6005783421175));
#33568=CARTESIAN_POINT('Ctrl Pts',(206.250989881508,5.17467697034661,-10.7448816986032));
#33569=CARTESIAN_POINT('Ctrl Pts',(206.290480932061,6.95147564889709,-9.88918505508886));
#33570=CARTESIAN_POINT('Ctrl Pts',(206.329971982613,8.51148314731673,-8.58333556315843));
#33571=CARTESIAN_POINT('Ctrl Pts',(206.369463033166,9.66651554827986,-6.98485802456189));
#33572=CARTESIAN_POINT('Ctrl Pts',(206.408954083719,10.821547949243,-5.38638048596536));
#33573=CARTESIAN_POINT('Ctrl Pts',(206.448445134272,11.5716052527496,-3.49527490070271));
#33574=CARTESIAN_POINT('Ctrl Pts',(206.487936184825,11.8262079436201,-1.5396655943414));
#33575=CARTESIAN_POINT('Ctrl Pts',(206.527427235377,12.0808106344906,0.415943712019895));
#33576=CARTESIAN_POINT('Ctrl Pts',(206.56691828593,11.839958712725,2.43605673947986));
#33577=CARTESIAN_POINT('Ctrl Pts',(206.606409336483,11.1327061786376,4.27698697771965));
#33578=CARTESIAN_POINT('Ctrl Pts',(206.645900387036,10.4254536445503,6.11791721595947));
#33579=CARTESIAN_POINT('Ctrl Pts',(206.685391437588,9.25180049814112,7.77966466497909));
#33580=CARTESIAN_POINT('Ctrl Pts',(206.724882488141,7.75332467878485,9.06177250285198));
#33581=CARTESIAN_POINT('Ctrl Pts',(206.764373538694,6.25484885942861,10.3438803407248));
#33582=CARTESIAN_POINT('Ctrl Pts',(206.803864589247,4.43155036712525,11.246348567451));
#33583=CARTESIAN_POINT('Ctrl Pts',(206.8433556398,2.50337394814799,11.6603123175776));
#33584=CARTESIAN_POINT('Ctrl Pts',(206.882846690352,0.575197529170728,12.0742760677042));
#33585=CARTESIAN_POINT('Ctrl Pts',(206.922337740905,-1.45785681648046,11.9997353412312));
#33586=CARTESIAN_POINT('Ctrl Pts',(206.961828791458,-3.35054146531087,11.4456819961558));
#33587=CARTESIAN_POINT('Ctrl Pts',(207.001319842011,-5.24322611414129,10.8916286510803));
#33588=CARTESIAN_POINT('Ctrl Pts',(207.040810892563,-6.99554106615095,9.85806268740243));
#33589=CARTESIAN_POINT('Ctrl Pts',(207.080301943116,-8.39610432924578,8.46966330855321));
#33590=CARTESIAN_POINT('Ctrl Pts',(207.119792993669,-9.79666759234061,7.08126392970398));
#33591=CARTESIAN_POINT('Ctrl Pts',(207.159284044222,-10.8454791665206,5.33803113568344));
#33592=CARTESIAN_POINT('Ctrl Pts',(207.198775094774,-11.4160207682894,3.45025133661703));
#33593=CARTESIAN_POINT('Ctrl Pts',(207.222131114132,-11.7534536931892,2.33376998417775));
#33594=CARTESIAN_POINT('Ctrl Pts',(207.24548713349,-11.9235953034982,1.16672836266624));
#33595=CARTESIAN_POINT('Ctrl Pts',(207.268843152848,-11.9241429677904,-0.000156968565329558));
#33596=CARTESIAN_POINT('Origin',(212.6,0.,0.));
#33597=CARTESIAN_POINT('',(208.981156847152,-11.9250072207259,0.000301374860750547));
#33598=CARTESIAN_POINT('',(208.768843152848,-11.9248763938011,0.000301080366776068));
#33599=CARTESIAN_POINT('',(212.6,-11.925,-1.46039130798322E-15));
#33600=CARTESIAN_POINT('Ctrl Pts',(208.981156847152,-11.9250072207259,0.000301374860750547));
#33601=CARTESIAN_POINT('Ctrl Pts',(208.97203530728,-11.925467717682,0.455925961038745));
#33602=CARTESIAN_POINT('Ctrl Pts',(208.962913767407,-11.8998498269624,0.91149906648302));
#33603=CARTESIAN_POINT('Ctrl Pts',(208.953792227535,-11.8477510063931,1.36402344065116));
#33604=CARTESIAN_POINT('Ctrl Pts',(208.914301176982,-11.6221929114159,3.3231951580302));
#33605=CARTESIAN_POINT('Ctrl Pts',(208.87481012643,-10.9002776652053,5.2252216173048));
#33606=CARTESIAN_POINT('Ctrl Pts',(208.835319075877,-9.76909000255087,6.84066110680794));
#33607=CARTESIAN_POINT('Ctrl Pts',(208.795828025324,-8.63790233989649,8.45610059631109));
#33608=CARTESIAN_POINT('Ctrl Pts',(208.756336974771,-7.0974422607984,9.78495311604276));
#33609=CARTESIAN_POINT('Ctrl Pts',(208.716845924218,-5.33353567508007,10.666919004979));
#33610=CARTESIAN_POINT('Ctrl Pts',(208.677354873666,-3.5696290893617,11.5488848939153));
#33611=CARTESIAN_POINT('Ctrl Pts',(208.637863823113,-1.58227599702309,11.9839641520561));
#33612=CARTESIAN_POINT('Ctrl Pts',(208.59837277256,0.388788926863556,11.9196731090447));
#33613=CARTESIAN_POINT('Ctrl Pts',(208.558881722007,2.3598538507502,11.8553820660332));
#33614=CARTESIAN_POINT('Ctrl Pts',(208.519390671455,4.31463060618487,11.2917207218694));
#33615=CARTESIAN_POINT('Ctrl Pts',(208.479899620902,6.01731420606716,10.296683621516));
#33616=CARTESIAN_POINT('Ctrl Pts',(208.440408570349,7.71999780594943,9.30164652116268));
#33617=CARTESIAN_POINT('Ctrl Pts',(208.400917519796,9.17058825027933,7.87523366461978));
#33618=CARTESIAN_POINT('Ctrl Pts',(208.361426469244,10.1941006155549,6.18951342967102));
#33619=CARTESIAN_POINT('Ctrl Pts',(208.321935418691,11.2176129808304,4.50379319472225));
#33620=CARTESIAN_POINT('Ctrl Pts',(208.282444368138,11.8140472670516,2.55876558136763));
#33621=CARTESIAN_POINT('Ctrl Pts',(208.242953317585,11.9114555247774,0.589059536366358));
#33622=CARTESIAN_POINT('Ctrl Pts',(208.203462267032,12.0088637825032,-1.38064650863491));
#33623=CARTESIAN_POINT('Ctrl Pts',(208.16397121648,11.6072460117335,-3.37503098528282));
#33624=CARTESIAN_POINT('Ctrl Pts',(208.124480165927,10.7550494190316,-5.1535110216552));
#33625=CARTESIAN_POINT('Ctrl Pts',(208.084989115374,9.9028528263298,-6.93199105802757));
#33626=CARTESIAN_POINT('Ctrl Pts',(208.045498064821,8.60007741169578,-8.4945666541244));
#33627=CARTESIAN_POINT('Ctrl Pts',(208.006007014269,7.00387715140256,-9.65274410228489));
#33628=CARTESIAN_POINT('Ctrl Pts',(207.966515963716,5.40767689110933,-10.8109215504454));
#33629=CARTESIAN_POINT('Ctrl Pts',(207.927024913163,3.51805178515689,-11.5647008506695));
#33630=CARTESIAN_POINT('Ctrl Pts',(207.88753386261,1.56294756826656,-11.8231535029781));
#33631=CARTESIAN_POINT('Ctrl Pts',(207.848042812058,-0.39215664862377,-12.0816061552867));
#33632=CARTESIAN_POINT('Ctrl Pts',(207.808551761505,-2.41273997645199,-11.8447321596798));
#33633=CARTESIAN_POINT('Ctrl Pts',(207.769060710952,-4.25505917229834,-11.1411056586128));
#33634=CARTESIAN_POINT('Ctrl Pts',(207.729569660399,-6.09737836814469,-10.4374791575458));
#33635=CARTESIAN_POINT('Ctrl Pts',(207.690078609846,-7.76143343200917,-9.26710015101879));
#33636=CARTESIAN_POINT('Ctrl Pts',(207.650587559294,-9.04648917416844,-7.77115161850466));
#33637=CARTESIAN_POINT('Ctrl Pts',(207.611096508741,-10.3315449163277,-6.27520308599052));
#33638=CARTESIAN_POINT('Ctrl Pts',(207.571605458188,-11.2376013367818,-4.45368502748925));
#33639=CARTESIAN_POINT('Ctrl Pts',(207.532114407635,-11.6553607257316,-2.52632741528232));
#33640=CARTESIAN_POINT('Ctrl Pts',(207.515128554141,-11.8350470009086,-1.69733417316286));
#33641=CARTESIAN_POINT('Ctrl Pts',(207.498142700646,-11.9243971510314,-0.848760359091592));
#33642=CARTESIAN_POINT('Ctrl Pts',(207.481156847152,-11.9240882605208,-0.000122447896127587));
#33643=CARTESIAN_POINT('Ctrl Pts',(207.268843152848,-11.9241429677904,-0.000156968565329558));
#33644=CARTESIAN_POINT('Ctrl Pts',(207.284978184043,-11.9245213105338,-0.806275979334776));
#33645=CARTESIAN_POINT('Ctrl Pts',(207.301113215238,-11.8439616826702,-1.61232040125019));
#33646=CARTESIAN_POINT('Ctrl Pts',(207.317248246433,-11.6817049171041,-2.40156921564886));
#33647=CARTESIAN_POINT('Ctrl Pts',(207.356739296986,-11.2845758347925,-4.33328316473606));
#33648=CARTESIAN_POINT('Ctrl Pts',(207.396230347538,-10.3980460408117,-6.1643842587982));
#33649=CARTESIAN_POINT('Ctrl Pts',(207.435721398091,-9.12905774534167,-7.67398652266591));
#33650=CARTESIAN_POINT('Ctrl Pts',(207.475212448644,-7.86006944987165,-9.18358878653363));
#33651=CARTESIAN_POINT('Ctrl Pts',(207.514703499197,-6.20862265291245,-10.3716922202069));
#33652=CARTESIAN_POINT('Ctrl Pts',(207.554194549749,-4.37393160722762,-11.0949757441439));
#33653=CARTESIAN_POINT('Ctrl Pts',(207.593685600302,-2.53924056154279,-11.8182592680808));
#33654=CARTESIAN_POINT('Ctrl Pts',(207.633176650855,-0.521305267132348,
-12.0767228822814));
#33655=CARTESIAN_POINT('Ctrl Pts',(207.672667701408,1.43645046571683,-11.8391880856495));
#33656=CARTESIAN_POINT('Ctrl Pts',(207.712158751961,3.39420619856601,-11.6016532890176));
#33657=CARTESIAN_POINT('Ctrl Pts',(207.751649802513,5.29178236985393,-10.8681200815533));
#33658=CARTESIAN_POINT('Ctrl Pts',(207.791140853066,6.90027410676151,-9.7270746742996));
#33659=CARTESIAN_POINT('Ctrl Pts',(207.830631903619,8.50876584366908,-8.58602926704593));
#33660=CARTESIAN_POINT('Ctrl Pts',(207.870122954172,9.8281731461963,-7.03747166000294));
#33661=CARTESIAN_POINT('Ctrl Pts',(207.909614004724,10.6993357311611,-5.26820456889654));
#33662=CARTESIAN_POINT('Ctrl Pts',(207.949105055277,11.570498316126,-3.49893747779013));
#33663=CARTESIAN_POINT('Ctrl Pts',(207.98859610583,11.9934161835284,-1.5089609026203));
#33664=CARTESIAN_POINT('Ctrl Pts',(208.028087156383,11.9170726932381,0.461674010448334));
#33665=CARTESIAN_POINT('Ctrl Pts',(208.067578206935,11.8407292029477,2.43230892351694));
#33666=CARTESIAN_POINT('Ctrl Pts',(208.107069257488,11.2651243549645,4.38360217448438));
#33667=CARTESIAN_POINT('Ctrl Pts',(208.146560308041,10.2596934407489,6.08016899187007));
#33668=CARTESIAN_POINT('Ctrl Pts',(208.186051358594,9.25426252653324,7.77673580925578));
#33669=CARTESIAN_POINT('Ctrl Pts',(208.225542409147,7.81900554608517,9.21857619305974));
#33670=CARTESIAN_POINT('Ctrl Pts',(208.265033459699,6.12705774506347,10.2317607407768));
#33671=CARTESIAN_POINT('Ctrl Pts',(208.304524510252,4.4351099440418,11.2449452884938));
#33672=CARTESIAN_POINT('Ctrl Pts',(208.344015560805,2.48647132244651,11.829474000124));
#33673=CARTESIAN_POINT('Ctrl Pts',(208.383506611358,0.516206423454282,11.9148350973158));
#33674=CARTESIAN_POINT('Ctrl Pts',(208.422997661911,-1.45405847553796,12.0001961945076));
#33675=CARTESIAN_POINT('Ctrl Pts',(208.462488712463,-3.44594965192712,11.5863896772611));
#33676=CARTESIAN_POINT('Ctrl Pts',(208.501979763016,-5.21918500094195,10.7233330822924));
#33677=CARTESIAN_POINT('Ctrl Pts',(208.541470813569,-6.9924203499568,9.86027648732369));
#33678=CARTESIAN_POINT('Ctrl Pts',(208.580961864122,-8.5469998715973,8.54796981463284));
#33679=CARTESIAN_POINT('Ctrl Pts',(208.620452914674,-9.69539442575685,6.94471679745451));
#33680=CARTESIAN_POINT('Ctrl Pts',(208.659943965227,-10.8437889799164,5.34146378027619));
#33681=CARTESIAN_POINT('Ctrl Pts',(208.69943501578,-11.585998566595,3.44726441861042));
#33682=CARTESIAN_POINT('Ctrl Pts',(208.738926066333,-11.8324903419393,1.49061624027016));
#33683=CARTESIAN_POINT('Ctrl Pts',(208.748898428504,-11.894734957408,0.996519375179027));
#33684=CARTESIAN_POINT('Ctrl Pts',(208.758870790676,-11.9253689368238,0.49844031140405));
#33685=CARTESIAN_POINT('Ctrl Pts',(208.768843152848,-11.9248763938011,0.000301080366776068));
#33686=CARTESIAN_POINT('Origin',(212.6,0.,0.));
#33687=CARTESIAN_POINT('',(210.481156847152,-11.9257187659321,-0.000199934177370631));
#33688=CARTESIAN_POINT('',(210.268843152848,-11.9258152927569,-0.000165876011026085));
#33689=CARTESIAN_POINT('',(212.6,-11.925,-1.46039130798322E-15));
#33690=CARTESIAN_POINT('Ctrl Pts',(210.481156847152,-11.9257187659321,-0.000199934177370631));
#33691=CARTESIAN_POINT('Ctrl Pts',(210.445927913913,-11.9243221171086,1.75919632918402));
#33692=CARTESIAN_POINT('Ctrl Pts',(210.410698980674,-11.5299628057005,3.51919798316331));
#33693=CARTESIAN_POINT('Ctrl Pts',(210.375470047435,-10.7763254526979,5.108872047103));
#33694=CARTESIAN_POINT('Ctrl Pts',(210.335978996882,-9.93151046485828,6.8908703379858));
#33695=CARTESIAN_POINT('Ctrl Pts',(210.296487946329,-8.63522530351655,8.45883432193996));
#33696=CARTESIAN_POINT('Ctrl Pts',(210.256996895776,-7.04384102480421,9.6236202893412));
#33697=CARTESIAN_POINT('Ctrl Pts',(210.217505845224,-5.45245674609186,10.7884062567424));
#33698=CARTESIAN_POINT('Ctrl Pts',(210.178014794671,-3.56597335000889,11.5500142075908));
#33699=CARTESIAN_POINT('Ctrl Pts',(210.138523744118,-1.61195758638579,11.8165712707125));
#33700=CARTESIAN_POINT('Ctrl Pts',(210.099032693566,0.342058177237336,12.0831283338342));
#33701=CARTESIAN_POINT('Ctrl Pts',(210.059541643013,2.3636063084006,11.8546345092293));
#33702=CARTESIAN_POINT('Ctrl Pts',(210.02005059246,4.20882717982609,11.1586530381804));
#33703=CARTESIAN_POINT('Ctrl Pts',(209.980559541907,6.05404805125158,10.4626715671314));
#33704=CARTESIAN_POINT('Ctrl Pts',(209.941068491354,7.7229416629393,9.29920244963827));
#33705=CARTESIAN_POINT('Ctrl Pts',(209.901577440802,9.01418915048089,7.8085951243157));
#33706=CARTESIAN_POINT('Ctrl Pts',(209.862086390249,10.3054366380225,6.31798779899315));
#33707=CARTESIAN_POINT('Ctrl Pts',(209.822595339696,11.2190380014179,4.50024226584114));
#33708=CARTESIAN_POINT('Ctrl Pts',(209.783104289143,11.6447853833703,2.57463341689275));
#33709=CARTESIAN_POINT('Ctrl Pts',(209.743613238591,12.0705327653226,0.649024567944349));
#33710=CARTESIAN_POINT('Ctrl Pts',(209.704122188038,12.0084261658319,-1.38444759680043));
#33711=CARTESIAN_POINT('Ctrl Pts',(209.664631137485,11.4659575124806,-3.2804850522635));
#33712=CARTESIAN_POINT('Ctrl Pts',(209.625140086932,10.9234888591293,-5.17652250772661));
#33713=CARTESIAN_POINT('Ctrl Pts',(209.58564903638,9.90065815191745,-6.93512525390801));
#33714=CARTESIAN_POINT('Ctrl Pts',(209.546157985827,8.52084959881122,-8.34415280124789));
#33715=CARTESIAN_POINT('Ctrl Pts',(209.506666935274,7.14104104570499,-9.75318034858777));
#33716=CARTESIAN_POINT('Ctrl Pts',(209.467175884721,5.40425464670437,-10.8126326970861));
#33717=CARTESIAN_POINT('Ctrl Pts',(209.427684834168,3.51999918242787,-11.3947079651846));
#33718=CARTESIAN_POINT('Ctrl Pts',(209.388193783616,1.63574371815139,-11.9767832332831));
#33719=CARTESIAN_POINT('Ctrl Pts',(209.348702733063,-0.395980811400968,
-12.0814814209816));
#33720=CARTESIAN_POINT('Ctrl Pts',(209.30921168251,-2.33008719862318,-11.6961727715927));
#33721=CARTESIAN_POINT('Ctrl Pts',(209.269720631957,-4.26419358584538,-11.3108641222038));
#33722=CARTESIAN_POINT('Ctrl Pts',(209.230229581405,-6.10068183073744,-10.4355486357274));
#33723=CARTESIAN_POINT('Ctrl Pts',(209.190738530852,-7.61801610538814,-9.17581573889653));
#33724=CARTESIAN_POINT('Ctrl Pts',(209.151247480299,-9.13535038003885,-7.91608284206565));
#33725=CARTESIAN_POINT('Ctrl Pts',(209.111756429746,-10.3335306844482,-6.27193253488027));
#33726=CARTESIAN_POINT('Ctrl Pts',(209.072265379193,-11.0680203647811,-4.44169889354584));
#33727=CARTESIAN_POINT('Ctrl Pts',(209.041895868513,-11.6328595341468,-3.03420784581842));
#33728=CARTESIAN_POINT('Ctrl Pts',(209.011526357832,-11.9234740292446,-1.51666790116677));
#33729=CARTESIAN_POINT('Ctrl Pts',(208.981156847152,-11.9250072207259,0.000301374860750547));
#33730=CARTESIAN_POINT('Ctrl Pts',(208.768843152848,-11.9248763938011,0.000301080366776068));
#33731=CARTESIAN_POINT('Ctrl Pts',(208.798361841229,-11.9234184419388,-1.47421583728277));
#33732=CARTESIAN_POINT('Ctrl Pts',(208.82788052961,-11.6492331794196,-2.94925993414675));
#33733=CARTESIAN_POINT('Ctrl Pts',(208.857399217991,-11.1148764047439,-4.32311079838467));
#33734=CARTESIAN_POINT('Ctrl Pts',(208.896890268544,-10.3999967281943,-6.16109266368449));
#33735=CARTESIAN_POINT('Ctrl Pts',(208.936381319096,-9.21946341108495,-7.81795939926939));
#33736=CARTESIAN_POINT('Ctrl Pts',(208.975872369649,-7.71568434876186,-9.09384294443857));
#33737=CARTESIAN_POINT('Ctrl Pts',(209.015363420202,-6.21190528643878,-10.3697264896077));
#33738=CARTESIAN_POINT('Ctrl Pts',(209.054854470755,-4.38488047890197,-11.2646268443612));
#33739=CARTESIAN_POINT('Ctrl Pts',(209.094345521308,-2.45500417832141,-11.6705920566297));
#33740=CARTESIAN_POINT('Ctrl Pts',(209.13383657186,-0.525127877740846,-12.0765572688982));
#33741=CARTESIAN_POINT('Ctrl Pts',(209.173327622413,1.50759991588345,-11.9935873386817));
#33742=CARTESIAN_POINT('Ctrl Pts',(209.212818672966,3.39797097106338,-11.431690939999));
#33743=CARTESIAN_POINT('Ctrl Pts',(209.252309723519,5.28834202624329,-10.8697945413162));
#33744=CARTESIAN_POINT('Ctrl Pts',(209.291800774071,7.03635634297882,-9.82897167416715));
#33745=CARTESIAN_POINT('Ctrl Pts',(209.331291824624,8.43115071540099,-8.43477694322957));
#33746=CARTESIAN_POINT('Ctrl Pts',(209.370782875177,9.82594508782317,-7.04058221229198));
#33747=CARTESIAN_POINT('Ctrl Pts',(209.41027392573,10.867519515932,-5.29301561756582));
#33748=CARTESIAN_POINT('Ctrl Pts',(209.449764976283,11.4302287341484,-3.402886356153));
#33749=CARTESIAN_POINT('Ctrl Pts',(209.489256026835,11.9929379523648,-1.51275709474018));
#33750=CARTESIAN_POINT('Ctrl Pts',(209.528747077388,12.0767819606888,0.519934833359339));
#33751=CARTESIAN_POINT('Ctrl Pts',(209.568238127941,11.6716466449402,2.44998552312061));
#33752=CARTESIAN_POINT('Ctrl Pts',(209.607729178494,11.2665113291916,4.38003621288187));
#33753=CARTESIAN_POINT('Ctrl Pts',(209.647220229046,10.3723966893704,6.20744566430488));
#33754=CARTESIAN_POINT('Ctrl Pts',(209.686711279599,9.09715989664615,7.71177322557509));
#33755=CARTESIAN_POINT('Ctrl Pts',(209.726202330152,7.82192310392194,9.21610078684532));
#33756=CARTESIAN_POINT('Ctrl Pts',(209.765693380705,6.16556415829473,10.3973464579627));
#33757=CARTESIAN_POINT('Ctrl Pts',(209.805184431257,4.32788986569333,11.1130164122201));
#33758=CARTESIAN_POINT('Ctrl Pts',(209.84467548181,2.49021557309193,11.8286863664774));
#33759=CARTESIAN_POINT('Ctrl Pts',(209.884166532363,0.471225933516344,12.0787806038747));
#33760=CARTESIAN_POINT('Ctrl Pts',(209.923657582916,-1.48552805694534,11.8331302223829));
#33761=CARTESIAN_POINT('Ctrl Pts',(209.963148633469,-3.44228204740699,11.5874798408911));
#33762=CARTESIAN_POINT('Ctrl Pts',(210.002639684021,-5.33680038875474,10.8460848405102));
#33763=CARTESIAN_POINT('Ctrl Pts',(210.042130734574,-6.94054707461293,9.69837980143724));
#33764=CARTESIAN_POINT('Ctrl Pts',(210.081621785127,-8.54429376047112,8.55067476236425));
#33765=CARTESIAN_POINT('Ctrl Pts',(210.12111283568,-9.85726879083975,6.99665968459916));
#33766=CARTESIAN_POINT('Ctrl Pts',(210.160603886232,-10.7210878084062,5.22379561930672));
#33767=CARTESIAN_POINT('Ctrl Pts',(210.196683641771,-11.5102888690802,3.60407415878444));
#33768=CARTESIAN_POINT('Ctrl Pts',(210.23276339731,-11.9245799369333,1.80167970713185));
#33769=CARTESIAN_POINT('Ctrl Pts',(210.268843152848,-11.9258152927569,-0.000165876011026086));
#33770=CARTESIAN_POINT('Origin',(212.6,0.,0.));
#33771=CARTESIAN_POINT('',(211.981156847152,-11.9240555281102,-9.42862044917003E-5));
#33772=CARTESIAN_POINT('',(211.768843152848,-11.9240993487478,-0.000130385428097346));
#33773=CARTESIAN_POINT('',(212.6,-11.925,-1.46039130798322E-15));
#33774=CARTESIAN_POINT('Ctrl Pts',(211.981156847152,-11.9240555281102,-9.42862044917003E-5));
#33775=CARTESIAN_POINT('Ctrl Pts',(211.959311571099,-11.9237506840456,1.09133601012478));
#33776=CARTESIAN_POINT('Ctrl Pts',(211.937466295046,-11.7751872270301,2.18284765302012));
#33777=CARTESIAN_POINT('Ctrl Pts',(211.915621018993,-11.4794611311497,3.23291447374606));
#33778=CARTESIAN_POINT('Ctrl Pts',(211.87612996844,-10.9448588595244,5.13118491906222));
#33779=CARTESIAN_POINT('Ctrl Pts',(211.836638917888,-9.92932880492338,6.89401360690861));
#33780=CARTESIAN_POINT('Ctrl Pts',(211.797147867335,-8.55537449659076,8.30875027180494));
#33781=CARTESIAN_POINT('Ctrl Pts',(211.757656816782,-7.18142018825815,9.72348693670128));
#33782=CARTESIAN_POINT('Ctrl Pts',(211.718165766229,-5.44904162619398,10.7901315786476));
#33783=CARTESIAN_POINT('Ctrl Pts',(211.678674715676,-3.56721587304484,11.3800147087441));
#33784=CARTESIAN_POINT('Ctrl Pts',(211.639183665124,-1.68539011989571,11.9698978388406));
#33785=CARTESIAN_POINT('Ctrl Pts',(211.599692614571,0.345882824338399,12.0830194570873));
#33786=CARTESIAN_POINT('Ctrl Pts',(211.560201564018,2.28157022685008,11.7057336872187));
#33787=CARTESIAN_POINT('Ctrl Pts',(211.520710513465,4.2172576293617,11.32844791735));
#33788=CARTESIAN_POINT('Ctrl Pts',(211.481219462913,6.0573594901509,10.4607547593661));
#33789=CARTESIAN_POINT('Ctrl Pts',(211.44172841236,7.57990407032705,9.20732415747235));
#33790=CARTESIAN_POINT('Ctrl Pts',(211.402237361807,9.10244865050324,7.95389355557854));
#33791=CARTESIAN_POINT('Ctrl Pts',(211.362746311254,10.3074359500664,6.31472550977488));
#33792=CARTESIAN_POINT('Ctrl Pts',(211.323255260701,11.0495081864258,4.48755308539555));
#33793=CARTESIAN_POINT('Ctrl Pts',(211.283764210149,11.7915804227853,2.66038066101622));
#33794=CARTESIAN_POINT('Ctrl Pts',(211.244273159596,12.0707375959411,0.645203858061226));
#33795=CARTESIAN_POINT('Ctrl Pts',(211.204782109043,11.8533049379526,-1.31488627038385));
#33796=CARTESIAN_POINT('Ctrl Pts',(211.16529105849,11.6358722799641,-3.27497639882889));
#33797=CARTESIAN_POINT('Ctrl Pts',(211.125800007938,10.9218497908313,-5.17997985276401));
#33798=CARTESIAN_POINT('Ctrl Pts',(211.086308957385,9.79737010097926,-6.80009580524951));
#33799=CARTESIAN_POINT('Ctrl Pts',(211.046817906832,8.67289041112725,-8.42021175773503));
#33800=CARTESIAN_POINT('Ctrl Pts',(211.007326856279,7.137953520556,-9.75544020877092));
#33801=CARTESIAN_POINT('Ctrl Pts',(210.967835805727,5.37771907610233,-10.6447123678688));
#33802=CARTESIAN_POINT('Ctrl Pts',(210.928344755174,3.61748463164866,-11.5339845269667));
#33803=CARTESIAN_POINT('Ctrl Pts',(210.888853704621,1.63195263331257,-11.9773003941266));
#33804=CARTESIAN_POINT('Ctrl Pts',(210.849362654068,-0.339361922652062,
-11.9211827157203));
#33805=CARTESIAN_POINT('Ctrl Pts',(210.809871603515,-2.31067647861667,-11.8650650373139));
#33806=CARTESIAN_POINT('Ctrl Pts',(210.770380552962,-4.26777359220982,-11.3095138133413));
#33807=CARTESIAN_POINT('Ctrl Pts',(210.73088950241,-5.97456837120942,-10.3215452638584));
#33808=CARTESIAN_POINT('Ctrl Pts',(210.691398451857,-7.68136315020902,-9.33357671437552));
#33809=CARTESIAN_POINT('Ctrl Pts',(210.651907401304,-9.13785559461506,-7.91319083938231));
#33810=CARTESIAN_POINT('Ctrl Pts',(210.612416350752,-10.16834882185,-6.23172898105467));
#33811=CARTESIAN_POINT('Ctrl Pts',(210.572925300199,-11.1988420490849,-4.55026712272701));
#33812=CARTESIAN_POINT('Ctrl Pts',(210.533434249646,-11.8033360591487,-2.6077292810649));
#33813=CARTESIAN_POINT('Ctrl Pts',(210.493943199093,-11.9089106570118,-0.638444061328108));
#33814=CARTESIAN_POINT('Ctrl Pts',(210.489681081779,-11.9203049176139,-0.42590667593657));
#33815=CARTESIAN_POINT('Ctrl Pts',(210.485418964466,-11.9258877373027,-0.213057735605563));
#33816=CARTESIAN_POINT('Ctrl Pts',(210.481156847152,-11.9257187659321,-0.000199934177370631));
#33817=CARTESIAN_POINT('Ctrl Pts',(210.268843152848,-11.9258152927569,-0.000165876011026086));
#33818=CARTESIAN_POINT('Ctrl Pts',(210.272254447862,-11.9259320940794,-0.17052808502141));
#33819=CARTESIAN_POINT('Ctrl Pts',(210.275665742877,-11.9223563995277,-0.340885387442564));
#33820=CARTESIAN_POINT('Ctrl Pts',(210.279077037891,-11.9150559677764,-0.511082921451824));
#33821=CARTESIAN_POINT('Ctrl Pts',(210.318568088444,-11.830542104816,-2.48138434409818));
#33822=CARTESIAN_POINT('Ctrl Pts',(210.358059138996,-11.2468513741308,-4.43027413657111));
#33823=CARTESIAN_POINT('Ctrl Pts',(210.397550189549,-10.2343944683165,-6.12265745691662));
#33824=CARTESIAN_POINT('Ctrl Pts',(210.437041240102,-9.22193756250219,-7.81504077726213));
#33825=CARTESIAN_POINT('Ctrl Pts',(210.476532290655,-7.78071448155873,-9.25091762548023));
#33826=CARTESIAN_POINT('Ctrl Pts',(210.516023341207,-6.08458016266289,-10.2570779811783));
#33827=CARTESIAN_POINT('Ctrl Pts',(210.55551439176,-4.38844584376707,-11.2632383368764));
#33828=CARTESIAN_POINT('Ctrl Pts',(210.595005442313,-2.43740028691886,-11.8396822000545));
#33829=CARTESIAN_POINT('Ctrl Pts',(210.634496492866,-0.466798384223374,
-11.9168730687345));
#33830=CARTESIAN_POINT('Ctrl Pts',(210.673987543418,1.50380351847213,-11.9940639374146));
#33831=CARTESIAN_POINT('Ctrl Pts',(210.713478593971,3.49396176701487,-11.5720018115967));
#33832=CARTESIAN_POINT('Ctrl Pts',(210.752969644524,5.26360329995653,-10.7016001031869));
#33833=CARTESIAN_POINT('Ctrl Pts',(210.792460695077,7.0332448328982,-9.83119839477717));
#33834=CARTESIAN_POINT('Ctrl Pts',(210.831951745629,8.58236965023875,-8.51245710377558));
#33835=CARTESIAN_POINT('Ctrl Pts',(210.871442796182,9.72410661359659,-6.90445617230285));
#33836=CARTESIAN_POINT('Ctrl Pts',(210.910933846735,10.8658435769544,-5.29645524083012));
#33837=CARTESIAN_POINT('Ctrl Pts',(210.950424897288,11.6001926863296,-3.39919466888623));
#33838=CARTESIAN_POINT('Ctrl Pts',(210.989915947841,11.8385693083198,-1.44154125849834));
#33839=CARTESIAN_POINT('Ctrl Pts',(211.029406998393,12.07694593031,0.516112151889512));
#33840=CARTESIAN_POINT('Ctrl Pts',(211.068898048946,11.8193500649152,2.53415840072137));
#33841=CARTESIAN_POINT('Ctrl Pts',(211.108389099499,11.0968555365749,4.36916029326344));
#33842=CARTESIAN_POINT('Ctrl Pts',(211.147880150052,10.3743610082346,6.20416218580552));
#33843=CARTESIAN_POINT('Ctrl Pts',(211.187371200604,9.18696781694879,7.85611972205781));
#33844=CARTESIAN_POINT('Ctrl Pts',(211.226862251157,7.67791136562249,9.12575703870582));
#33845=CARTESIAN_POINT('Ctrl Pts',(211.26635330171,6.16885491429619,10.3953943553538));
#33846=CARTESIAN_POINT('Ctrl Pts',(211.305844352263,4.33813520292946,11.2827114523975));
#33847=CARTESIAN_POINT('Ctrl Pts',(211.345335402816,2.40659220044616,11.6806711471814));
#33848=CARTESIAN_POINT('Ctrl Pts',(211.384826453368,0.475049197962844,12.0786308419652));
#33849=CARTESIAN_POINT('Ctrl Pts',(211.424317503921,-1.55731709563709,11.9872331344892));
#33850=CARTESIAN_POINT('Ctrl Pts',(211.463808554474,-3.44534205666278,11.4175033426943));
#33851=CARTESIAN_POINT('Ctrl Pts',(211.503299605027,-5.3333670176885,10.8477735508993));
#33852=CARTESIAN_POINT('Ctrl Pts',(211.542790655579,-7.07705064613995,9.79971167478558));
#33853=CARTESIAN_POINT('Ctrl Pts',(211.582281706132,-8.46605214766769,8.3997455616712));
#33854=CARTESIAN_POINT('Ctrl Pts',(211.621772756685,-9.85505364919538,6.99977944855687));
#33855=CARTESIAN_POINT('Ctrl Pts',(211.661263807238,-10.8893730237993,5.24790909844197));
#33856=CARTESIAN_POINT('Ctrl Pts',(211.700754857791,-11.4442401839961,3.35546287102892));
#33857=CARTESIAN_POINT('Ctrl Pts',(211.723450956143,-11.7631306532074,2.26784567414334));
#33858=CARTESIAN_POINT('Ctrl Pts',(211.746147054496,-11.9236593462382,1.13379664328528));
#33859=CARTESIAN_POINT('Ctrl Pts',(211.768843152848,-11.9240993487478,-0.000130385428097346));
#33860=CARTESIAN_POINT('Origin',(212.6,0.,0.));
#33861=CARTESIAN_POINT('',(213.481156847152,-11.9251100366554,0.000297839544098621));
#33862=CARTESIAN_POINT('',(213.268843152848,-11.9249776593072,0.000301781866272833));
#33863=CARTESIAN_POINT('',(212.6,-11.925,-1.46039130798322E-15));
#33864=CARTESIAN_POINT('Ctrl Pts',(213.481156847152,-11.9251100366554,0.000297839544098621));
#33865=CARTESIAN_POINT('Ctrl Pts',(213.472695228285,-11.925539783909,0.422948611961856));
#33866=CARTESIAN_POINT('Ctrl Pts',(213.464233609418,-11.9035018557077,0.84555479724396));
#33867=CARTESIAN_POINT('Ctrl Pts',(213.455771990551,-11.8586550796965,1.26572649372693));
#33868=CARTESIAN_POINT('Ctrl Pts',(213.416280939998,-11.649351596942,3.22670133407911));
#33869=CARTESIAN_POINT('Ctrl Pts',(213.376789889446,-10.9432341408314,5.13464903060221));
#33870=CARTESIAN_POINT('Ctrl Pts',(213.337298838893,-9.82548175657631,6.75941359197088));
#33871=CARTESIAN_POINT('Ctrl Pts',(213.29780778834,-8.70772937232116,8.38417815333963));
#33872=CARTESIAN_POINT('Ctrl Pts',(213.258316737787,-7.17834205992146,9.72575957955392));
#33873=CARTESIAN_POINT('Ctrl Pts',(213.218825687234,-5.4218100198409,10.6223227198616));
#33874=CARTESIAN_POINT('Ctrl Pts',(213.179334636682,-3.66527797976036,11.5188858601692));
#33875=CARTESIAN_POINT('Ctrl Pts',(213.139843586129,-1.68160121199899,11.9704307145702));
#33876=CARTESIAN_POINT('Ctrl Pts',(213.100352535576,0.289929083907081,11.922487365581));
#33877=CARTESIAN_POINT('Ctrl Pts',(213.060861485023,2.26145937981309,11.8745440165919));
#33878=CARTESIAN_POINT('Ctrl Pts',(213.021370434471,4.22084320386379,11.3271124642125));
#33879=CARTESIAN_POINT('Ctrl Pts',(212.981879383918,5.93171981764215,10.3462294514053));
#33880=CARTESIAN_POINT('Ctrl Pts',(212.942388333365,7.64259643142056,9.36534643859798));
#33881=CARTESIAN_POINT('Ctrl Pts',(212.902897282812,9.1049658349266,7.95101196536274));
#33882=CARTESIAN_POINT('Ctrl Pts',(212.86340623226,10.1424222072035,6.27383739245451));
#33883=CARTESIAN_POINT('Ctrl Pts',(212.823915181707,11.1798785794803,4.59666281954626));
#33884=CARTESIAN_POINT('Ctrl Pts',(212.784424131154,11.792421920528,2.65664814696501));
#33885=CARTESIAN_POINT('Ctrl Pts',(212.744933080601,11.9061610434206,0.687817609739553));
#33886=CARTESIAN_POINT('Ctrl Pts',(212.705442030048,12.0199001663132,-1.28101292748585));
#33887=CARTESIAN_POINT('Ctrl Pts',(212.665950979496,11.6348350710507,-3.27865932935547));
#33888=CARTESIAN_POINT('Ctrl Pts',(212.626459928943,10.7974162126884,-5.06414523746193));
#33889=CARTESIAN_POINT('Ctrl Pts',(212.58696887839,9.95999735432603,-6.84963114556838));
#33890=CARTESIAN_POINT('Ctrl Pts',(212.547477827837,8.67022473286378,-8.42295655991168));
#33891=CARTESIAN_POINT('Ctrl Pts',(212.507986777285,7.08368379585762,-9.59433102078714));
#33892=CARTESIAN_POINT('Ctrl Pts',(212.468495726732,5.49714285885149,-10.7657054816626));
#33893=CARTESIAN_POINT('Ctrl Pts',(212.429004676179,3.61383360630147,-11.5351289890702));
#33894=CARTESIAN_POINT('Ctrl Pts',(212.389513625626,1.66093989066995,-11.8097858801807));
#33895=CARTESIAN_POINT('Ctrl Pts',(212.350022575074,-0.291953824961641,
-12.0844427712912));
#33896=CARTESIAN_POINT('Ctrl Pts',(212.310531524521,-2.31443200367473,-11.8643330461045));
#33897=CARTESIAN_POINT('Ctrl Pts',(212.271040473968,-4.16252282642839,-11.1760085708448));
#33898=CARTESIAN_POINT('Ctrl Pts',(212.231549423415,-6.01061364918205,-10.4876840955851));
#33899=CARTESIAN_POINT('Ctrl Pts',(212.192058372862,-7.68431711597629,-9.33114487025232));
#33900=CARTESIAN_POINT('Ctrl Pts',(212.15256732231,-8.98173414892402,-7.84590437962295));
#33901=CARTESIAN_POINT('Ctrl Pts',(212.113076271757,-10.2791511818717,-6.36066388899365));
#33902=CARTESIAN_POINT('Ctrl Pts',(212.073585221204,-11.2002817809729,-4.54672213306777));
#33903=CARTESIAN_POINT('Ctrl Pts',(212.034094170651,-11.6340098361987,-2.6228951537119));
#33904=CARTESIAN_POINT('Ctrl Pts',(212.016448396151,-11.8278124155081,-1.7632721105357));
#33905=CARTESIAN_POINT('Ctrl Pts',(211.998802621652,-11.9243017694307,-0.881709736823186));
#33906=CARTESIAN_POINT('Ctrl Pts',(211.981156847152,-11.9240555281102,-9.42862044917003E-5));
#33907=CARTESIAN_POINT('Ctrl Pts',(211.768843152848,-11.9240993487478,-0.000130385428097346));
#33908=CARTESIAN_POINT('Ctrl Pts',(211.785638105048,-11.9244249474918,-0.839228363854304));
#33909=CARTESIAN_POINT('Ctrl Pts',(211.802433057249,-11.8370876556473,-1.67825953518361));
#33910=CARTESIAN_POINT('Ctrl Pts',(211.819228009449,-11.6613877061497,-2.49835970882992));
#33911=CARTESIAN_POINT('Ctrl Pts',(211.858719060002,-11.248253122317,-4.42671395656453));
#33912=CARTESIAN_POINT('Ctrl Pts',(211.898210110554,-10.3465690088622,-6.25040034732254));
#33913=CARTESIAN_POINT('Ctrl Pts',(211.937701161107,-9.06510564359358,-7.74942734260614));
#33914=CARTESIAN_POINT('Ctrl Pts',(211.97719221166,-7.78364227832489,-9.24845433788976));
#33915=CARTESIAN_POINT('Ctrl Pts',(212.016683262213,-6.12239966124234,-10.4228219376989));
#33916=CARTESIAN_POINT('Ctrl Pts',(212.056174312765,-4.28177371622964,-11.1308660180082));
#33917=CARTESIAN_POINT('Ctrl Pts',(212.095665363318,-2.44114777121695,-11.8389100983174));
#33918=CARTESIAN_POINT('Ctrl Pts',(212.135156413871,-0.421138498274144,
-12.0806306591266));
#33919=CARTESIAN_POINT('Ctrl Pts',(212.174647464424,1.5345801079983,-11.8268689161578));
#33920=CARTESIAN_POINT('Ctrl Pts',(212.214138514977,3.49029871427071,-11.573107173189));
#33921=CARTESIAN_POINT('Ctrl Pts',(212.253629565529,5.38172665387273,-10.8238631264422));
#33922=CARTESIAN_POINT('Ctrl Pts',(212.293120616082,6.98070071601359,-9.66951818764984));
#33923=CARTESIAN_POINT('Ctrl Pts',(212.332611666635,8.57967477815445,-8.51517324885752));
#33924=CARTESIAN_POINT('Ctrl Pts',(212.372102717188,9.88619496283413,-6.95572741801974));
#33925=CARTESIAN_POINT('Ctrl Pts',(212.41159376774,10.7426555616574,-5.17929685878644));
#33926=CARTESIAN_POINT('Ctrl Pts',(212.451084818293,11.5991161604807,-3.40286629955314));
#33927=CARTESIAN_POINT('Ctrl Pts',(212.490575868846,12.0055171734476,-1.40945101192424));
#33928=CARTESIAN_POINT('Ctrl Pts',(212.530066919399,11.9128343908349,0.560483045581709));
#33929=CARTESIAN_POINT('Ctrl Pts',(212.569557969951,11.8201516082223,2.53041710308769));
#33930=CARTESIAN_POINT('Ctrl Pts',(212.609049020504,11.2283850300301,4.47686993047078));
#33931=CARTESIAN_POINT('Ctrl Pts',(212.648540071057,10.2089195394423,6.16504065720881));
#33932=CARTESIAN_POINT('Ctrl Pts',(212.68803112161,9.18945404885441,7.85321138394682));
#33933=CARTESIAN_POINT('Ctrl Pts',(212.727522172163,7.74228964587083,9.28310001003975));
#33934=CARTESIAN_POINT('Ctrl Pts',(212.767013222715,6.04199797015777,10.2822188751482));
#33935=CARTESIAN_POINT('Ctrl Pts',(212.806504273268,4.34170629444471,11.2813377402566));
#33936=CARTESIAN_POINT('Ctrl Pts',(212.845995323821,2.38828734600218,11.8496868443805));
#33937=CARTESIAN_POINT('Ctrl Pts',(212.885486374374,0.417382319487588,11.9187061574327));
#33938=CARTESIAN_POINT('Ctrl Pts',(212.924977424926,-1.55352270702703,11.9877254704848));
#33939=CARTESIAN_POINT('Ctrl Pts',(212.964468475479,-3.5419138116137,11.5574149924652));
#33940=CARTESIAN_POINT('Ctrl Pts',(213.003959526032,-5.3079311036409,10.679683135133));
#33941=CARTESIAN_POINT('Ctrl Pts',(213.043450576585,-7.07394839566808,9.80195127780094));
#33942=CARTESIAN_POINT('Ctrl Pts',(213.082941627138,-8.61759187513578,8.47679804115636));
#33943=CARTESIAN_POINT('Ctrl Pts',(213.12243267769,-9.75265161819899,6.86407684119899));
#33944=CARTESIAN_POINT('Ctrl Pts',(213.161923728243,-10.8877113612622,5.2513556412416));
#33945=CARTESIAN_POINT('Ctrl Pts',(213.201414778796,-11.614187367921,3.35106647797142));
#33946=CARTESIAN_POINT('Ctrl Pts',(213.240905829349,-11.8444447382294,1.3924414928011));
#33947=CARTESIAN_POINT('Ctrl Pts',(213.250218270515,-11.8987420583598,0.930575331067063));
#33948=CARTESIAN_POINT('Ctrl Pts',(213.259530711682,-11.9254461332588,0.465465287460084));
#33949=CARTESIAN_POINT('Ctrl Pts',(213.268843152848,-11.9249776593072,0.000301781866272833));
#33950=CARTESIAN_POINT('Origin',(212.6,0.,0.));
#33951=CARTESIAN_POINT('',(214.981156847152,-11.9256350387103,-0.000223418725388003));
#33952=CARTESIAN_POINT('',(214.768843152848,-11.92574165171,-0.000192647346739548));
#33953=CARTESIAN_POINT('',(212.6,-11.925,-1.46039130798322E-15));
#33954=CARTESIAN_POINT('Ctrl Pts',(214.981156847152,-11.9256350387103,-0.000223418725388003));
#33955=CARTESIAN_POINT('Ctrl Pts',(214.946587834918,-11.9241468048938,1.72625030866615));
#33956=CARTESIAN_POINT('Ctrl Pts',(214.912018822685,-11.5448800822796,3.45335664987414));
#33957=CARTESIAN_POINT('Ctrl Pts',(214.877449810451,-10.8183213363969,5.01933136170478));
#33958=CARTESIAN_POINT('Ctrl Pts',(214.837958759898,-9.98831300496768,6.80827418978669));
#33959=CARTESIAN_POINT('Ctrl Pts',(214.798467709345,-8.70507509800421,8.38693398487368));
#33960=CARTESIAN_POINT('Ctrl Pts',(214.758976658793,-7.12340477955964,9.56487680018312));
#33961=CARTESIAN_POINT('Ctrl Pts',(214.71948560824,-5.54173446111503,10.7428196154926));
#33962=CARTESIAN_POINT('Ctrl Pts',(214.679994557687,-3.66163173118932,11.5200454510245));
#33963=CARTESIAN_POINT('Ctrl Pts',(214.640503507134,-1.70989363898263,11.8027974480418));
#33964=CARTESIAN_POINT('Ctrl Pts',(214.601012456582,0.241844453224007,12.085549445059));
#33965=CARTESIAN_POINT('Ctrl Pts',(214.561521406029,2.26521790771161,11.8738276035617));
#33966=CARTESIAN_POINT('Ctrl Pts',(214.522030355476,4.11614690820027,11.1931719582184));
#33967=CARTESIAN_POINT('Ctrl Pts',(214.482539304923,5.96707590868894,10.5125163128752));
#33968=CARTESIAN_POINT('Ctrl Pts',(214.44304825437,7.64556045517865,9.36292686368587));
#33969=CARTESIAN_POINT('Ctrl Pts',(214.403557203818,8.94912472748544,7.88307874298126));
#33970=CARTESIAN_POINT('Ctrl Pts',(214.364066153265,10.2526889997922,6.40323062227666));
#33971=CARTESIAN_POINT('Ctrl Pts',(214.324575102712,11.1813329979161,4.59312383005675));
#33972=CARTESIAN_POINT('Ctrl Pts',(214.285084052159,11.6230342694774,2.67111179599225));
#33973=CARTESIAN_POINT('Ctrl Pts',(214.245593001607,12.0647355410387,0.749099761927715));
#33974=CARTESIAN_POINT('Ctrl Pts',(214.206101951054,12.0194940860374,-1.28481751398142));
#33975=CARTESIAN_POINT('Ctrl Pts',(214.166610900501,11.492767387372,-3.18528831283648));
#33976=CARTESIAN_POINT('Ctrl Pts',(214.127119849948,10.9660406887066,-5.08575911169154));
#33977=CARTESIAN_POINT('Ctrl Pts',(214.087628799396,9.95782874637702,-6.85278343349253));
#33978=CARTESIAN_POINT('Ctrl Pts',(214.048137748843,8.58975230474426,-8.27320489286197));
#33979=CARTESIAN_POINT('Ctrl Pts',(214.00864669829,7.22167586311151,-9.69362635223138));
#33980=CARTESIAN_POINT('Ctrl Pts',(213.969155647737,5.49373492217559,-10.7674449491692));
#33981=CARTESIAN_POINT('Ctrl Pts',(213.929664597184,3.61437123374004,-11.365125799605));
#33982=CARTESIAN_POINT('Ctrl Pts',(213.890173546632,1.73500754530452,-11.9628066500407));
#33983=CARTESIAN_POINT('Ctrl Pts',(213.850682496079,-0.295778890630705,
-12.0843497539743));
#33984=CARTESIAN_POINT('Ctrl Pts',(213.811191445526,-2.23301402882067,-11.7150933501712));
#33985=CARTESIAN_POINT('Ctrl Pts',(213.771700394973,-4.17024916701075,-11.345836946368));
#33986=CARTESIAN_POINT('Ctrl Pts',(213.732209344421,-6.01393300745556,-10.485781034828));
#33987=CARTESIAN_POINT('Ctrl Pts',(213.692718293868,-7.54166171656932,-9.23867427767465));
#33988=CARTESIAN_POINT('Ctrl Pts',(213.653227243315,-9.06939042568303,-7.99156752052131));
#33989=CARTESIAN_POINT('Ctrl Pts',(213.613736192762,-10.2811640034656,-6.35740991775461));
#33990=CARTESIAN_POINT('Ctrl Pts',(213.57424514221,-11.0308060376576,-4.5333301242806));
#33991=CARTESIAN_POINT('Ctrl Pts',(213.543215710524,-11.61982471311,-3.10008997115947));
#33992=CARTESIAN_POINT('Ctrl Pts',(213.512186278838,-11.9235341191794,-1.54959627362695));
#33993=CARTESIAN_POINT('Ctrl Pts',(213.481156847152,-11.9251100366554,0.000297839544098621));
#33994=CARTESIAN_POINT('Ctrl Pts',(213.268843152848,-11.9249776593072,0.000301781866272833));
#33995=CARTESIAN_POINT('Ctrl Pts',(213.299021762234,-11.9234594867745,-1.50714266637844));
#33996=CARTESIAN_POINT('Ctrl Pts',(213.329200371621,-11.6365756334932,-3.01514857156817));
#33997=CARTESIAN_POINT('Ctrl Pts',(213.359378981007,-11.0786438839662,-4.41513467066438));
#33998=CARTESIAN_POINT('Ctrl Pts',(213.39887003156,-10.3485469254364,-6.24712504188916));
#33999=CARTESIAN_POINT('Ctrl Pts',(213.438361082112,-9.15431427441883,-7.89414497726828));
#34000=CARTESIAN_POINT('Ctrl Pts',(213.477852132665,-7.64000637878046,-9.15751423695523));
#34001=CARTESIAN_POINT('Ctrl Pts',(213.517343183218,-6.12569848314209,-10.4208834966422));
#34002=CARTESIAN_POINT('Ctrl Pts',(213.556834233771,-4.29131534288294,-11.3006020806369));
#34003=CARTESIAN_POINT('Ctrl Pts',(213.596325284324,-2.35813884685473,-11.6905494159513));
#34004=CARTESIAN_POINT('Ctrl Pts',(213.635816334876,-0.424962350826485,
-12.0804967512656));
#34005=CARTESIAN_POINT('Ctrl Pts',(213.675307385429,1.60700750097082,-11.9806728378995));
#34006=CARTESIAN_POINT('Ctrl Pts',(213.714798435982,3.49265390767523,-11.4031194481618));
#34007=CARTESIAN_POINT('Ctrl Pts',(213.754289486535,5.37830031437964,-10.825566058424));
#34008=CARTESIAN_POINT('Ctrl Pts',(213.793780537087,7.11762327599115,-9.77028319231473));
#34009=CARTESIAN_POINT('Ctrl Pts',(213.83327158764,8.50080802599692,-8.36456976616193));
#34010=CARTESIAN_POINT('Ctrl Pts',(213.872762638193,9.88399277600267,-6.95885634000915));
#34011=CARTESIAN_POINT('Ctrl Pts',(213.912253688746,10.9110393144027,-5.20271235381288));
#34012=CARTESIAN_POINT('Ctrl Pts',(213.951744739298,11.4580548769386,-3.30798169657998));
#34013=CARTESIAN_POINT('Ctrl Pts',(213.991235789851,12.0050704394744,-1.41325103934708));
#34014=CARTESIAN_POINT('Ctrl Pts',(214.030726840404,12.0720550261461,0.620066288922465));
#34015=CARTESIAN_POINT('Ctrl Pts',(214.070217890957,11.650928277111,2.54669094109573));
#34016=CARTESIAN_POINT('Ctrl Pts',(214.10970894151,11.2298015280759,4.473315593269));
#34017=CARTESIAN_POINT('Ctrl Pts',(214.149199992062,10.3205634433338,6.29324756934605));
#34018=CARTESIAN_POINT('Ctrl Pts',(214.188691042615,9.03289553728178,7.78694822638488));
#34019=CARTESIAN_POINT('Ctrl Pts',(214.228182093168,7.74522763122972,9.28064888342373));
#34020=CARTESIAN_POINT('Ctrl Pts',(214.267673143721,6.07912990386763,10.4481182214244));
#34021=CARTESIAN_POINT('Ctrl Pts',(214.307164194273,4.23558395169564,11.1485242546259));
#34022=CARTESIAN_POINT('Ctrl Pts',(214.346655244826,2.39203799952365,11.8489302878274));
#34023=CARTESIAN_POINT('Ctrl Pts',(214.386146295379,0.371043822541859,12.0822730162297));
#34024=CARTESIAN_POINT('Ctrl Pts',(214.425637345932,-1.5836057755406,11.8204042746227));
#34025=CARTESIAN_POINT('Ctrl Pts',(214.465128396485,-3.53825537362304,11.5585355330157));
#34026=CARTESIAN_POINT('Ctrl Pts',(214.504619447037,-5.42656039280606,10.8014553213994));
#34027=CARTESIAN_POINT('Ctrl Pts',(214.54411049759,-7.02073434061572,9.64049032914524));
#34028=CARTESIAN_POINT('Ctrl Pts',(214.583601548143,-8.6149082884254,8.47952533689109));
#34029=CARTESIAN_POINT('Ctrl Pts',(214.623092598696,-9.9149511648617,6.9146755639991));
#34030=CARTESIAN_POINT('Ctrl Pts',(214.662583649248,-10.7640386201078,5.13470905238759));
#34031=CARTESIAN_POINT('Ctrl Pts',(214.698003483782,-11.5255918517417,3.53824305734485));
#34032=CARTESIAN_POINT('Ctrl Pts',(214.733423318315,-11.9243768133226,1.76872774634368));
#34033=CARTESIAN_POINT('Ctrl Pts',(214.768843152848,-11.92574165171,-0.000192647346739548));
#34034=CARTESIAN_POINT('Origin',(212.6,0.,0.));
#34035=CARTESIAN_POINT('',(216.481156847152,-11.9240315088021,-6.52149305474525E-5));
#34036=CARTESIAN_POINT('',(216.268843152848,-11.9240641358096,-0.000102538611651484));
#34037=CARTESIAN_POINT('',(212.6,-11.925,-1.46039130798322E-15));
#34038=CARTESIAN_POINT('Ctrl Pts',(216.481156847152,-11.9240315088021,-6.52149305474525E-5));
#34039=CARTESIAN_POINT('Ctrl Pts',(216.459971492104,-11.9238275369958,1.05840031273444));
#34040=CARTESIAN_POINT('Ctrl Pts',(216.438786137057,-11.7842138861413,2.11691862153893));
#34041=CARTESIAN_POINT('Ctrl Pts',(216.417600782009,-11.5058760523776,3.13760738835481));
#34042=CARTESIAN_POINT('Ctrl Pts',(216.378109731456,-10.9870339825039,5.04024586660471));
#34043=CARTESIAN_POINT('Ctrl Pts',(216.338618680904,-9.98615748628875,6.81143544251588));
#34044=CARTESIAN_POINT('Ctrl Pts',(216.299127630351,-8.62398243222592,8.23751727553837));
#34045=CARTESIAN_POINT('Ctrl Pts',(216.259636579798,-7.26180737816309,9.66359910856087));
#34046=CARTESIAN_POINT('Ctrl Pts',(216.220145529245,-5.53833376625262,10.7445731986947));
#34047=CARTESIAN_POINT('Ctrl Pts',(216.180654478692,-3.66146445378734,11.3500414937473));
#34048=CARTESIAN_POINT('Ctrl Pts',(216.14116342814,-1.7845951413221,11.9555097888));
#34049=CARTESIAN_POINT('Ctrl Pts',(216.101672377587,0.245669871697946,12.0854722887714));
#34050=CARTESIAN_POINT('Ctrl Pts',(216.062181327034,2.18441943934548,11.7242515995327));
#34051=CARTESIAN_POINT('Ctrl Pts',(216.022690276481,4.12316900699302,11.3630309102939));
#34052=CARTESIAN_POINT('Ctrl Pts',(215.983199225929,5.97040312926806,10.5106270318449));
#34053=CARTESIAN_POINT('Ctrl Pts',(215.943708175376,7.50328970160239,9.26986556051175));
#34054=CARTESIAN_POINT('Ctrl Pts',(215.904217124823,9.03617627393673,8.02910408917863));
#34055=CARTESIAN_POINT('Ctrl Pts',(215.86472607427,10.2547152963304,6.39998502496138));
#34056=CARTESIAN_POINT('Ctrl Pts',(215.825235023717,11.011914240016,4.57902922317239));
#34057=CARTESIAN_POINT('Ctrl Pts',(215.785743973165,11.7691131837017,2.7580734213834));
#34058=CARTESIAN_POINT('Ctrl Pts',(215.746252922612,12.0649720486793,0.745280882022666));
#34059=CARTESIAN_POINT('Ctrl Pts',(215.706761872059,11.8638013396419,-1.21654495586739));
#34060=CARTESIAN_POINT('Ctrl Pts',(215.667270821506,11.6626306306044,-3.17837079375747));
#34061=CARTESIAN_POINT('Ctrl Pts',(215.627779770954,10.9644303475518,-5.08922993017687));
#34062=CARTESIAN_POINT('Ctrl Pts',(215.588288720401,9.85342448602773,-6.7186151664077));
#34063=CARTESIAN_POINT('Ctrl Pts',(215.548797669848,8.7424186245037,-8.34800040263853));
#34064=CARTESIAN_POINT('Ctrl Pts',(215.509306619295,7.21860718450825,-9.6959117386808));
#34065=CARTESIAN_POINT('Ctrl Pts',(215.469815568742,5.46580774825511,-10.5997504458949));
#34066=CARTESIAN_POINT('Ctrl Pts',(215.43032451819,3.713008312002,-11.503589153109));
#34067=CARTESIAN_POINT('Ctrl Pts',(215.390833467637,1.73122087949119,-11.9633552314949));
#34068=CARTESIAN_POINT('Ctrl Pts',(215.351342417084,-0.240491260510576,
-11.9235870361965));
#34069=CARTESIAN_POINT('Ctrl Pts',(215.311851366531,-2.21220340051235,-11.8838188408981));
#34070=CARTESIAN_POINT('Ctrl Pts',(215.272360315979,-4.17384024800508,-11.3445163719153));
#34071=CARTESIAN_POINT('Ctrl Pts',(215.232869265426,-5.88876928204609,-10.3707357597696));
#34072=CARTESIAN_POINT('Ctrl Pts',(215.193378214873,-7.60369831608712,-9.39695514762394));
#34073=CARTESIAN_POINT('Ctrl Pts',(215.15388716432,-9.07191953667642,-7.98869639231527));
#34074=CARTESIAN_POINT('Ctrl Pts',(215.114396113767,-10.1163212173628,-6.31583793991495));
#34075=CARTESIAN_POINT('Ctrl Pts',(215.074905063215,-11.1607228980492,-4.64297948751464));
#34076=CARTESIAN_POINT('Ctrl Pts',(215.035414012662,-11.7813050388328,-2.70552133802269));
#34077=CARTESIAN_POINT('Ctrl Pts',(214.995922962109,-11.903206731277,-0.737179332738295));
#34078=CARTESIAN_POINT('Ctrl Pts',(214.99100092379,-11.9184001685996,-0.491851476438355));
#34079=CARTESIAN_POINT('Ctrl Pts',(214.986078885471,-11.9258469378476,-0.246043860042586));
#34080=CARTESIAN_POINT('Ctrl Pts',(214.981156847152,-11.9256350387103,-0.000223418725388003));
#34081=CARTESIAN_POINT('Ctrl Pts',(214.768843152848,-11.92574165171,-0.000192647346739548));
#34082=CARTESIAN_POINT('Ctrl Pts',(214.772914368868,-11.9258985285555,-0.203515365788062));
#34083=CARTESIAN_POINT('Ctrl Pts',(214.776985584887,-11.920804851864,-0.406830224423079));
#34084=CARTESIAN_POINT('Ctrl Pts',(214.781056800907,-11.9104080006084,-0.609873533518392));
#34085=CARTESIAN_POINT('Ctrl Pts',(214.820547851459,-11.809557891807,-2.57940635748183));
#34086=CARTESIAN_POINT('Ctrl Pts',(214.860038902012,-11.2097256401482,-4.52338875507772));
#34087=CARTESIAN_POINT('Ctrl Pts',(214.899529952565,-10.183269092108,-6.20731786406665));
#34088=CARTESIAN_POINT('Ctrl Pts',(214.939021003118,-9.15681254406792,-7.89124697305558));
#34089=CARTESIAN_POINT('Ctrl Pts',(214.978512053671,-7.70373169964654,-9.31512279343753));
#34090=CARTESIAN_POINT('Ctrl Pts',(215.018003104223,-5.99931189964917,-10.3071829904476));
#34091=CARTESIAN_POINT('Ctrl Pts',(215.057494154776,-4.2948920996518,-11.2992431874576));
#34092=CARTESIAN_POINT('Ctrl Pts',(215.096985205329,-2.33913334407844,-11.8594877610957));
#34093=CARTESIAN_POINT('Ctrl Pts',(215.136476255882,-0.367959078840414,
-11.9203343318945));
#34094=CARTESIAN_POINT('Ctrl Pts',(215.175967306434,1.60321518639762,-11.9811809026933));
#34095=CARTESIAN_POINT('Ctrl Pts',(215.215458356987,3.58980496130032,-11.5426294706528));
#34096=CARTESIAN_POINT('Ctrl Pts',(215.25494940754,5.35216764988208,-10.6575825549418));
#34097=CARTESIAN_POINT('Ctrl Pts',(215.294440458093,7.11453033846384,-9.7725356392308));
#34098=CARTESIAN_POINT('Ctrl Pts',(215.333931508646,8.65266594072465,-8.44099323984933));
#34099=CARTESIAN_POINT('Ctrl Pts',(215.373422559198,9.78102894879953,-6.82357949837102));
#34100=CARTESIAN_POINT('Ctrl Pts',(215.412913609751,10.9093919568744,-5.20616575689267));
#34101=CARTESIAN_POINT('Ctrl Pts',(215.452404660304,11.6279823707634,-3.30288067331745));
#34102=CARTESIAN_POINT('Ctrl Pts',(215.491895710857,11.8501165306539,-1.34331778733379));
#34103=CARTESIAN_POINT('Ctrl Pts',(215.531386761409,12.0722506905443,0.616245098649828));
#34104=CARTESIAN_POINT('Ctrl Pts',(215.570877811962,11.7979285964363,2.63208578704189));
#34105=CARTESIAN_POINT('Ctrl Pts',(215.610368862515,11.0602417600243,4.46103314016583));
#34106=CARTESIAN_POINT('Ctrl Pts',(215.649859913068,10.3225549236123,6.28998049328975));
#34107=CARTESIAN_POINT('Ctrl Pts',(215.68935096362,9.12150334489629,7.93203451114556));
#34108=CARTESIAN_POINT('Ctrl Pts',(215.728842014173,7.60197003992331,9.18911399319609));
#34109=CARTESIAN_POINT('Ctrl Pts',(215.768333064726,6.08243673495028,10.4461934752467));
#34110=CARTESIAN_POINT('Ctrl Pts',(215.807824115279,4.2444217037202,11.318298421492));
#34111=CARTESIAN_POINT('Ctrl Pts',(215.847315165832,2.30964495058899,11.7002266931057));
#34112=CARTESIAN_POINT('Ctrl Pts',(215.886806216384,0.374868197457755,12.0821549647194));
#34113=CARTESIAN_POINT('Ctrl Pts',(215.926297266937,-1.65667027757459,11.9739065617016));
#34114=CARTESIAN_POINT('Ctrl Pts',(215.96578831749,-3.53990571068435,11.3885395036988));
#34115=CARTESIAN_POINT('Ctrl Pts',(216.005279368043,-5.42314114379405,10.8031724456961));
#34116=CARTESIAN_POINT('Ctrl Pts',(216.044770418595,-7.15807353498107,9.74068673270843));
#34117=CARTESIAN_POINT('Ctrl Pts',(216.084261469148,-8.53541775284281,8.3292501614671));
#34118=CARTESIAN_POINT('Ctrl Pts',(216.123752519701,-9.91276197070455,6.91781359022576));
#34119=CARTESIAN_POINT('Ctrl Pts',(216.163243570254,-10.932518015241,5.15742616073064));
#34120=CARTESIAN_POINT('Ctrl Pts',(216.202734620806,-11.4716725754646,3.26044364913367));
#34121=CARTESIAN_POINT('Ctrl Pts',(216.224770798154,-11.7725231565545,2.20191918688213));
#34122=CARTESIAN_POINT('Ctrl Pts',(216.246806975501,-11.9237294127371,1.10086327286869));
#34123=CARTESIAN_POINT('Ctrl Pts',(216.268843152848,-11.9240641358096,-0.000102538611651484));
#34124=CARTESIAN_POINT('Origin',(212.6,0.,0.));
#34125=CARTESIAN_POINT('',(217.981156847152,-11.9252129121757,0.000290991664972789));
#34126=CARTESIAN_POINT('',(217.768843152848,-11.9250802682536,0.000299202489012452));
#34127=CARTESIAN_POINT('',(212.6,-11.925,-1.46039130798322E-15));
#34128=CARTESIAN_POINT('Ctrl Pts',(217.981156847152,-11.9252129121757,0.000290991664972789));
#34129=CARTESIAN_POINT('Ctrl Pts',(217.97335514929,-11.9256075493655,0.389969574352947));
#34130=CARTESIAN_POINT('Ctrl Pts',(217.965553451429,-11.9068787673408,0.779610388074303));
#34131=CARTESIAN_POINT('Ctrl Pts',(217.957751753567,-11.8687436293108,1.16734250236723));
#34132=CARTESIAN_POINT('Ctrl Pts',(217.918260703014,-11.6757091526497,3.12998560879517));
#34133=CARTESIAN_POINT('Ctrl Pts',(217.878769652462,-10.9854380465733,5.04372333236306));
#34134=CARTESIAN_POINT('Ctrl Pts',(217.839278601909,-9.8811978089238,6.67770122999309));
#34135=CARTESIAN_POINT('Ctrl Pts',(217.799787551356,-8.7769575712744,8.31167912762302));
#34136=CARTESIAN_POINT('Ctrl Pts',(217.760296500803,-7.25874820205201,9.66589719931515));
#34137=CARTESIAN_POINT('Ctrl Pts',(217.720805450251,-5.50971150490726,10.5769959340461));
#34138=CARTESIAN_POINT('Ctrl Pts',(217.681314399698,-3.76067480776247,11.4880946687772));
#34139=CARTESIAN_POINT('Ctrl Pts',(217.641823349145,-1.78081078269529,11.956074066547));
#34140=CARTESIAN_POINT('Ctrl Pts',(217.602332298592,0.191049302430142,11.9244817086603));
#34141=CARTESIAN_POINT('Ctrl Pts',(217.562841248039,2.16290938755557,11.8928893507736));
#34142=CARTESIAN_POINT('Ctrl Pts',(217.523350197487,4.12676553273927,11.3617252372304));
#34143=CARTESIAN_POINT('Ctrl Pts',(217.483859146934,5.84571750285487,10.3950637676231));
#34144=CARTESIAN_POINT('Ctrl Pts',(217.444368096381,7.56466947297048,9.42840229801586));
#34145=CARTESIAN_POINT('Ctrl Pts',(217.404877045828,9.03871726801803,8.02624347234463));
#34146=CARTESIAN_POINT('Ctrl Pts',(217.365385995275,10.0900463010733,6.35772990133517));
#34147=CARTESIAN_POINT('Ctrl Pts',(217.325894944723,11.1413753341286,4.68921633032567));
#34148=CARTESIAN_POINT('Ctrl Pts',(217.28640389417,11.7699856051916,2.75434801397791));
#34149=CARTESIAN_POINT('Ctrl Pts',(217.246912843617,11.9000477713734,0.786528381665041));
#34150=CARTESIAN_POINT('Ctrl Pts',(217.207421793064,12.0301099375552,-1.18129125064785));
#34151=CARTESIAN_POINT('Ctrl Pts',(217.167930742512,11.6616239988558,-3.18206219892579));
#34152=CARTESIAN_POINT('Ctrl Pts',(217.128439691959,10.8390404644088,-4.97443119030136));
#34153=CARTESIAN_POINT('Ctrl Pts',(217.088948641406,10.0164569299618,-6.76680018167684));
#34154=CARTESIAN_POINT('Ctrl Pts',(217.049457590853,8.73977579976731,-8.35076721614989));
#34155=CARTESIAN_POINT('Ctrl Pts',(217.009966540301,7.16300329300085,-9.53525813392556));
#34156=CARTESIAN_POINT('Ctrl Pts',(216.970475489748,5.58623078623438,-10.7197490517012));
#34157=CARTESIAN_POINT('Ctrl Pts',(216.930984439195,3.70936690289596,-11.5047638527795));
#34158=CARTESIAN_POINT('Ctrl Pts',(216.891493388642,1.75881798967936,-11.7956060944453));
#34159=CARTESIAN_POINT('Ctrl Pts',(216.85200233809,-0.191730923537244,-12.0864483361111));
#34160=CARTESIAN_POINT('Ctrl Pts',(216.812511287537,-2.21596486663205,-11.8831180183643));
#34161=CARTESIAN_POINT('Ctrl Pts',(216.773020236984,-4.06970022246687,-11.210142905217));
#34162=CARTESIAN_POINT('Ctrl Pts',(216.733529186431,-5.92343557830169,-10.5371677920697));
#34163=CARTESIAN_POINT('Ctrl Pts',(216.694038135878,-7.60667234687653,-9.39454788352191));
#34164=CARTESIAN_POINT('Ctrl Pts',(216.654547085326,-8.91636144680795,-7.92011757526435));
#34165=CARTESIAN_POINT('Ctrl Pts',(216.615056034773,-10.2260505467394,-6.44568726700679));
#34166=CARTESIAN_POINT('Ctrl Pts',(216.57556498422,-11.1621919780274,-4.6394465590395));
#34167=CARTESIAN_POINT('Ctrl Pts',(216.536073933667,-11.6118588719053,-2.71928251476157));
#34168=CARTESIAN_POINT('Ctrl Pts',(216.517768238162,-11.8202976225301,-1.82920899626814));
#34169=CARTESIAN_POINT('Ctrl Pts',(216.499462542657,-11.924207755354,-0.914656809388016));
#34170=CARTESIAN_POINT('Ctrl Pts',(216.481156847152,-11.9240315088021,-6.52149305474525E-5));
#34171=CARTESIAN_POINT('Ctrl Pts',(216.268843152848,-11.9240641358096,-0.000102538611651484));
#34172=CARTESIAN_POINT('Ctrl Pts',(216.286298026054,-11.9243292702156,-0.872178413671098));
#34173=CARTESIAN_POINT('Ctrl Pts',(216.303752899259,-11.829934037933,-1.74419775627108));
#34174=CARTESIAN_POINT('Ctrl Pts',(216.321207772465,-11.6402685376495,-2.59497838897577));
#34175=CARTESIAN_POINT('Ctrl Pts',(216.360698823018,-11.2111568636999,-4.51984032178938));
#34176=CARTESIAN_POINT('Ctrl Pts',(216.40018987357,-10.2943804398899,-6.33598659371769));
#34177=CARTESIAN_POINT('Ctrl Pts',(216.439680924123,-9.00053013148815,-7.82433523182753));
#34178=CARTESIAN_POINT('Ctrl Pts',(216.479171974676,-7.70667982308639,-9.31268386993737));
#34179=CARTESIAN_POINT('Ctrl Pts',(216.518663025229,-6.03575563009282,-10.4732348742287));
#34180=CARTESIAN_POINT('Ctrl Pts',(216.558154075781,-4.18932136621622,-11.1659908184813));
#34181=CARTESIAN_POINT('Ctrl Pts',(216.597645126334,-2.34288710233966,-11.8587467627338));
#34182=CARTESIAN_POINT('Ctrl Pts',(216.637136176887,-0.320942767580052,
-12.0837076469475));
#34183=CARTESIAN_POINT('Ctrl Pts',(216.67662722744,1.63260421669074,-11.8137364089219));
#34184=CARTESIAN_POINT('Ctrl Pts',(216.716118277992,3.58615120096156,-11.5437651708964));
#34185=CARTESIAN_POINT('Ctrl Pts',(216.755609328545,5.47130083474357,-10.7788618106316));
#34186=CARTESIAN_POINT('Ctrl Pts',(216.795100379098,7.06064726013488,-9.61129672498948));
#34187=CARTESIAN_POINT('Ctrl Pts',(216.834591429651,8.64999368552619,-8.44373163934735));
#34188=CARTESIAN_POINT('Ctrl Pts',(216.874082480203,9.9435369025268,-6.87350482832784));
#34189=CARTESIAN_POINT('Ctrl Pts',(216.913573530756,10.7852366161257,-5.09003296669331));
#34190=CARTESIAN_POINT('Ctrl Pts',(216.953064581309,11.6269363297247,-3.30656110505875));
#34191=CARTESIAN_POINT('Ctrl Pts',(216.992555631862,12.0167925399219,-1.30984419280916));
#34192=CARTESIAN_POINT('Ctrl Pts',(217.032046682415,11.9077768388131,0.659253536107953));
#34193=CARTESIAN_POINT('Ctrl Pts',(217.071537732967,11.7987611377042,2.62835126502504));
#34194=CARTESIAN_POINT('Ctrl Pts',(217.11102878352,11.1908735252894,4.56982981060956));
#34195=CARTESIAN_POINT('Ctrl Pts',(217.150519834073,10.1574435673132,6.24948835063251));
#34196=CARTESIAN_POINT('Ctrl Pts',(217.190010884626,9.124013609337,7.9291468906555));
#34197=CARTESIAN_POINT('Ctrl Pts',(217.229501935179,7.66504130579948,9.34698542511683));
#34198=CARTESIAN_POINT('Ctrl Pts',(217.268992985731,5.9565226850241,10.331969897877));
#34199=CARTESIAN_POINT('Ctrl Pts',(217.308484036284,4.24800406424873,11.3169543706372));
#34200=CARTESIAN_POINT('Ctrl Pts',(217.347975086837,2.28993912623549,11.8690847816963));
#34201=CARTESIAN_POINT('Ctrl Pts',(217.38746613739,0.318529511998548,11.9217575641274));
#34202=CARTESIAN_POINT('Ctrl Pts',(217.426957187942,-1.65288010223834,11.9744303465586));
#34203=CARTESIAN_POINT('Ctrl Pts',(217.466448238495,-3.63763439269893,11.5276455003618));
#34204=CARTESIAN_POINT('Ctrl Pts',(217.505939289048,-5.39631217813664,10.6352987425807));
#34205=CARTESIAN_POINT('Ctrl Pts',(217.545430339601,-7.15498996357436,9.74295198479951));
#34206=CARTESIAN_POINT('Ctrl Pts',(217.584921390154,-8.68759124398921,8.40504331543394));
#34207=CARTESIAN_POINT('Ctrl Pts',(217.624412440706,-9.80923811751666,6.78296484007562));
#34208=CARTESIAN_POINT('Ctrl Pts',(217.663903491259,-10.9308849910441,5.16088636471731));
#34209=CARTESIAN_POINT('Ctrl Pts',(217.703394541812,-11.6415774576842,3.25463808336625));
#34210=CARTESIAN_POINT('Ctrl Pts',(217.742885592365,-11.8555845880801,1.29417098666344));
#34211=CARTESIAN_POINT('Ctrl Pts',(217.751538112526,-11.902473718262,0.864631107573521));
#34212=CARTESIAN_POINT('Ctrl Pts',(217.760190632687,-11.925519392479,0.432488445912876));
#34213=CARTESIAN_POINT('Ctrl Pts',(217.768843152848,-11.9250802682536,0.000299202489012452));
#34214=CARTESIAN_POINT('Origin',(212.6,0.,0.));
#34215=CARTESIAN_POINT('',(219.481156847152,-11.9255450374969,-0.000244099323242208));
#34216=CARTESIAN_POINT('',(219.268843152848,-11.9256599882878,-0.000216904810520898));
#34217=CARTESIAN_POINT('',(212.6,-11.925,-1.46039130798322E-15));
#34218=CARTESIAN_POINT('Ctrl Pts',(219.481156847152,-11.9255450374969,-0.000244099323242208));
#34219=CARTESIAN_POINT('Ctrl Pts',(219.447247755924,-11.9239920023089,1.69330829367419));
#34220=CARTESIAN_POINT('Ctrl Pts',(219.413338664695,-11.5594992250726,3.3875078677213));
#34221=CARTESIAN_POINT('Ctrl Pts',(219.379429573467,-10.8595732414316,4.929445496933));
#34222=CARTESIAN_POINT('Ctrl Pts',(219.339938522914,-10.0444286474036,6.72520983795926));
#34223=CARTESIAN_POINT('Ctrl Pts',(219.300447472361,-8.77432624161127,8.31445687564588));
#34224=CARTESIAN_POINT('Ctrl Pts',(219.260956421809,-7.20247865493554,9.50547553041038));
#34225=CARTESIAN_POINT('Ctrl Pts',(219.221465371256,-5.63063106825982,10.6964941851749));
#34226=CARTESIAN_POINT('Ctrl Pts',(219.181974320703,-3.75703830070067,11.4892844570173));
#34227=CARTESIAN_POINT('Ctrl Pts',(219.14248327015,-1.8077121018322,11.7882119434258));
#34228=CARTESIAN_POINT('Ctrl Pts',(219.102992219598,0.141614097036269,12.0871394298343));
#34229=CARTESIAN_POINT('Ctrl Pts',(219.063501169045,2.16667372721406,11.8922041308089));
#34230=CARTESIAN_POINT('Ctrl Pts',(219.024010118492,4.02318356787142,11.2269211198753));
#34231=CARTESIAN_POINT('Ctrl Pts',(218.984519067939,5.87969340852889,10.5616381089417));
#34232=CARTESIAN_POINT('Ctrl Pts',(218.945028017386,7.56765345966592,9.42600738609977));
#34233=CARTESIAN_POINT('Ctrl Pts',(218.905536966834,8.88344487013097,7.95702023976691));
#34234=CARTESIAN_POINT('Ctrl Pts',(218.866045916281,10.1992362805959,6.48803309343413));
#34235=CARTESIAN_POINT('Ctrl Pts',(218.826554865728,11.142859050389,4.68568952361048));
#34236=CARTESIAN_POINT('Ctrl Pts',(218.787063815175,11.6004838356406,2.76740648179358));
#34237=CARTESIAN_POINT('Ctrl Pts',(218.747572764623,12.0581086208923,0.849123439976685));
#34238=CARTESIAN_POINT('Ctrl Pts',(218.70808171407,12.0297354216026,-1.18509907383346));
#34239=CARTESIAN_POINT('Ctrl Pts',(218.668590663517,11.5187869007824,-3.08987252004248));
#34240=CARTESIAN_POINT('Ctrl Pts',(218.629099612964,11.0078383799622,-4.99464596625151));
#34241=CARTESIAN_POINT('Ctrl Pts',(218.589608562411,10.0143145376115,-6.76997034485942));
#34242=CARTESIAN_POINT('Ctrl Pts',(218.550117511859,8.65806429053415,-8.20168803340916));
#34243=CARTESIAN_POINT('Ctrl Pts',(218.510626461306,7.30181404345685,-9.63340572195891));
#34244=CARTESIAN_POINT('Ctrl Pts',(218.471135410753,5.58283739165299,-10.7215167204505));
#34245=CARTESIAN_POINT('Ctrl Pts',(218.4316443602,3.70849472352703,-11.3347620505055));
#34246=CARTESIAN_POINT('Ctrl Pts',(218.392153309648,1.83415205540107,-11.9480073805605));
#34247=CARTESIAN_POINT('Ctrl Pts',(218.352662259095,-0.195556629046985,
-12.0863870421789));
#34248=CARTESIAN_POINT('Ctrl Pts',(218.313171208542,-2.13578729389285,-11.7332082778509));
#34249=CARTESIAN_POINT('Ctrl Pts',(218.273680157989,-4.07601795873877,-11.3800295135228));
#34250=CARTESIAN_POINT('Ctrl Pts',(218.234189107437,-5.92677060398249,-10.5352923232482));
#34251=CARTESIAN_POINT('Ctrl Pts',(218.194698056884,-7.4647886851439,-9.30089746972142));
#34252=CARTESIAN_POINT('Ctrl Pts',(218.155207006331,-9.00280676630527,-8.06650261619464));
#34253=CARTESIAN_POINT('Ctrl Pts',(218.115715955778,-10.2280902833843,-6.44245009941565));
#34254=CARTESIAN_POINT('Ctrl Pts',(218.076224905225,-10.992833118301,-4.62464959638219));
#34255=CARTESIAN_POINT('Ctrl Pts',(218.044535552534,-11.6064963426142,-3.16596666805982));
#34256=CARTESIAN_POINT('Ctrl Pts',(218.012846199843,-11.9236099537796,-1.58252626966517));
#34257=CARTESIAN_POINT('Ctrl Pts',(217.981156847152,-11.9252129121757,0.000290991664972789));
#34258=CARTESIAN_POINT('Ctrl Pts',(217.768843152848,-11.9250802682536,0.000299202489012452));
#34259=CARTESIAN_POINT('Ctrl Pts',(217.79968168324,-11.9235151813752,-1.54007064004802));
#34260=CARTESIAN_POINT('Ctrl Pts',(217.830520213631,-11.6236255785851,-3.08103220501337));
#34261=CARTESIAN_POINT('Ctrl Pts',(217.861358744023,-11.0416494811308,-4.5068549126511));
#34262=CARTESIAN_POINT('Ctrl Pts',(217.900849794576,-10.2963854496338,-6.33272780320826));
#34263=CARTESIAN_POINT('Ctrl Pts',(217.940340845128,-9.08853559248812,-7.96978767226803));
#34264=CARTESIAN_POINT('Ctrl Pts',(217.979831895681,-7.56380300299659,-9.22055576414479));
#34265=CARTESIAN_POINT('Ctrl Pts',(218.019322946234,-6.03907041350506,-10.4713238560216));
#34266=CARTESIAN_POINT('Ctrl Pts',(218.058813996787,-4.19745509166771,-11.3358001707153));
#34267=CARTESIAN_POINT('Ctrl Pts',(218.098305047339,-2.26111134538818,-11.7097028122664));
#34268=CARTESIAN_POINT('Ctrl Pts',(218.137796097892,-0.324767599108595,
-12.0836054538175));
#34269=CARTESIAN_POINT('Ctrl Pts',(218.177287148445,1.70630457161319,-11.9669344222258));
#34270=CARTESIAN_POINT('Ctrl Pts',(218.216778198998,3.5870966533059,-11.3737637599735));
#34271=CARTESIAN_POINT('Ctrl Pts',(218.256269249551,5.46788873499856,-10.7805930977212));
#34272=CARTESIAN_POINT('Ctrl Pts',(218.295760300103,7.19840072766217,-9.71092280480824));
#34273=CARTESIAN_POINT('Ctrl Pts',(218.335251350656,8.56988073317214,-8.29378735482445));
#34274=CARTESIAN_POINT('Ctrl Pts',(218.374742401209,9.94136073868211,-6.87665190484067));
#34275=CARTESIAN_POINT('Ctrl Pts',(218.414233451762,10.9538087570385,-5.11205129778605));
#34276=CARTESIAN_POINT('Ctrl Pts',(218.453724502314,11.4850930454499,-3.21284954599589));
#34277=CARTESIAN_POINT('Ctrl Pts',(218.493215552867,12.0163773338614,-1.31364779420564));
#34278=CARTESIAN_POINT('Ctrl Pts',(218.53270660342,12.0664978923279,0.720155102320104));
#34279=CARTESIAN_POINT('Ctrl Pts',(218.572197653973,11.6294086710342,2.64322122228095));
#34280=CARTESIAN_POINT('Ctrl Pts',(218.611688704526,11.1923194497406,4.56628734224172));
#34281=CARTESIAN_POINT('Ctrl Pts',(218.651179755078,10.2680204486868,6.37861668563754));
#34282=CARTESIAN_POINT('Ctrl Pts',(218.690670805631,8.96800998266048,7.86158771615087));
#34283=CARTESIAN_POINT('Ctrl Pts',(218.730161856184,7.66799951663418,9.3445587466642));
#34284=CARTESIAN_POINT('Ctrl Pts',(218.769652906737,5.99227758563538,10.4981714642951));
#34285=CARTESIAN_POINT('Ctrl Pts',(218.809143957289,4.14298675516752,11.18326540928));
#34286=CARTESIAN_POINT('Ctrl Pts',(218.848635007842,2.29369592469966,11.8683593542649));
#34287=CARTESIAN_POINT('Ctrl Pts',(218.888126058395,0.270836194762722,12.0849345266039));
#34288=CARTESIAN_POINT('Ctrl Pts',(218.927617108948,-1.68157458903359,11.8068654336887));
#34289=CARTESIAN_POINT('Ctrl Pts',(218.9671081595,-3.6339853728299,11.5287963407735));
#34290=CARTESIAN_POINT('Ctrl Pts',(219.006599210053,-5.51594721048561,10.7560829826041));
#34291=CARTESIAN_POINT('Ctrl Pts',(219.046090260606,-7.10043878836543,9.5819378771089));
#34292=CARTESIAN_POINT('Ctrl Pts',(219.085581311159,-8.68493036624525,8.4077927716137));
#34293=CARTESIAN_POINT('Ctrl Pts',(219.125072361712,-9.97195168434919,6.83221591879273));
#34294=CARTESIAN_POINT('Ctrl Pts',(219.164563412264,-10.806249185254,5.04526936978167));
#34295=CARTESIAN_POINT('Ctrl Pts',(219.199323325792,-11.5405955392276,3.47240395715747));
#34296=CARTESIAN_POINT('Ctrl Pts',(219.23408323932,-11.9241953954151,1.73578046983011));
#34297=CARTESIAN_POINT('Ctrl Pts',(219.268843152848,-11.9256599882878,-0.000216904810520898));
#34298=CARTESIAN_POINT('Origin',(212.6,0.,0.));
#34299=CARTESIAN_POINT('',(220.981156847152,-11.9240411815327,1.80394148113772E-5));
#34300=CARTESIAN_POINT('',(220.768843152848,-11.9240373570162,-7.43698370121595E-5));
#34301=CARTESIAN_POINT('',(212.6,-11.925,-1.46039130798322E-15));
#34302=CARTESIAN_POINT('Ctrl Pts',(220.981156847152,-11.9240411815327,1.80394148113772E-5));
#34303=CARTESIAN_POINT('Ctrl Pts',(220.96063141311,-11.9239219583868,1.02549140231068));
#34304=CARTESIAN_POINT('Ctrl Pts',(220.940105979067,-11.7929513953952,2.05097956229081));
#34305=CARTESIAN_POINT('Ctrl Pts',(220.919580545025,-11.5314859766584,3.04206109250113));
#34306=CARTESIAN_POINT('Ctrl Pts',(220.880089494472,-11.0284250402679,4.94890753145148));
#34307=CARTESIAN_POINT('Ctrl Pts',(220.84059844392,-10.0422985541953,6.7283875893475));
#34308=CARTESIAN_POINT('Ctrl Pts',(220.801107393367,-8.6920036461207,8.16572986837976));
#34309=CARTESIAN_POINT('Ctrl Pts',(220.761616342814,-7.34170873804613,9.60307214741197));
#34310=CARTESIAN_POINT('Ctrl Pts',(220.722125292261,-5.62724540796957,10.6982766475804));
#34311=CARTESIAN_POINT('Ctrl Pts',(220.682634241708,-3.7554581716358,11.3192820256276));
#34312=CARTESIAN_POINT('Ctrl Pts',(220.643143191156,-1.88367093530202,11.9402874036747));
#34313=CARTESIAN_POINT('Ctrl Pts',(220.603652140603,0.145440207288969,12.0870936596005));
#34314=CARTESIAN_POINT('Ctrl Pts',(220.56416109005,2.08711696474266,11.7419659708025));
#34315=CARTESIAN_POINT('Ctrl Pts',(220.524670039497,4.02879372219635,11.3968382820046));
#34316=CARTESIAN_POINT('Ctrl Pts',(220.485178988944,5.88303609451274,10.559776648483));
#34317=CARTESIAN_POINT('Ctrl Pts',(220.445687938392,7.4261600300081,9.33176816120625));
#34318=CARTESIAN_POINT('Ctrl Pts',(220.406196887839,8.96928396550346,8.10375967392952));
#34319=CARTESIAN_POINT('Ctrl Pts',(220.366705837286,10.2012894641778,6.4848043328977));
#34320=CARTESIAN_POINT('Ctrl Pts',(220.327214786733,10.9735626651117,4.67019108695998));
#34321=CARTESIAN_POINT('Ctrl Pts',(220.287723736181,11.7458358660456,2.85557784102226));
#34322=CARTESIAN_POINT('Ctrl Pts',(220.248232685628,12.0583767692391,0.845306690178657));
#34323=CARTESIAN_POINT('Ctrl Pts',(220.208741635075,11.8734820243007,-1.11812027943816));
#34324=CARTESIAN_POINT('Ctrl Pts',(220.169250584522,11.6885872793624,-3.08154724905498));
#34325=CARTESIAN_POINT('Ctrl Pts',(220.12975953397,11.0062568862923,-4.998130037445));
#34326=CARTESIAN_POINT('Ctrl Pts',(220.090268483417,9.90880117091153,-6.63667234241024));
#34327=CARTESIAN_POINT('Ctrl Pts',(220.050777432864,8.81134545553077,-8.27521464737553));
#34328=CARTESIAN_POINT('Ctrl Pts',(220.011286382311,7.29876441783939,-9.63571646891601));
#34329=CARTESIAN_POINT('Ctrl Pts',(219.971795331758,5.55352057176231,-10.554059644325));
#34330=CARTESIAN_POINT('Ctrl Pts',(219.932304281206,3.80827672568522,-11.472402819734));
#34331=CARTESIAN_POINT('Ctrl Pts',(219.892813230653,1.83037007122243,-11.9485873490116));
#34332=CARTESIAN_POINT('Ctrl Pts',(219.8533221801,-0.141604077312892,-11.92517133466));
#34333=CARTESIAN_POINT('Ctrl Pts',(219.813831129547,-2.11357822584816,-11.9017553203085));
#34334=CARTESIAN_POINT('Ctrl Pts',(219.774340078995,-4.07961986845595,-11.3787387623278));
#34335=CARTESIAN_POINT('Ctrl Pts',(219.734849028442,-5.80256521181501,-10.4192130724648));
#34336=CARTESIAN_POINT('Ctrl Pts',(219.695357977889,-7.52551055517407,-9.45968738260177));
#34337=CARTESIAN_POINT('Ctrl Pts',(219.655866927336,-9.00535959928439,-8.06365256085633));
#34338=CARTESIAN_POINT('Ctrl Pts',(219.616375876784,-10.063597914105,-6.39951254893597));
#34339=CARTESIAN_POINT('Ctrl Pts',(219.576884826231,-11.1218362289256,-4.73537253701557));
#34340=CARTESIAN_POINT('Ctrl Pts',(219.537393775678,-11.7584638144564,-2.80312733492023));
#34341=CARTESIAN_POINT('Ctrl Pts',(219.497902725125,-11.8966842160899,-0.83586391168958));
#34342=CARTESIAN_POINT('Ctrl Pts',(219.492320765801,-11.9162213175072,-0.557796241793535));
#34343=CARTESIAN_POINT('Ctrl Pts',(219.486738806476,-11.925800691038,-0.279028939291055));
#34344=CARTESIAN_POINT('Ctrl Pts',(219.481156847152,-11.9255450374969,-0.000244099323242208));
#34345=CARTESIAN_POINT('Ctrl Pts',(219.268843152848,-11.9256599882878,-0.000216904810520898));
#34346=CARTESIAN_POINT('Ctrl Pts',(219.273574289873,-11.9258593325571,-0.236501769201835));
#34347=CARTESIAN_POINT('Ctrl Pts',(219.278305426898,-11.9189793690461,-0.472775034442688));
#34348=CARTESIAN_POINT('Ctrl Pts',(219.283036563923,-11.9049409507008,-0.708622204330391));
#34349=CARTESIAN_POINT('Ctrl Pts',(219.322527614475,-11.787761531537,-2.67725098423027));
#34350=CARTESIAN_POINT('Ctrl Pts',(219.362018665028,-11.1718290095037,-4.61619229882879));
#34351=CARTESIAN_POINT('Ctrl Pts',(219.401509715581,-10.1314434090349,-6.2915513919816));
#34352=CARTESIAN_POINT('Ctrl Pts',(219.441000766134,-9.09105780856628,-7.96691048513431));
#34353=CARTESIAN_POINT('Ctrl Pts',(219.480491816687,-7.62621912966225,-9.37868735684133));
#34354=CARTESIAN_POINT('Ctrl Pts',(219.519982867239,-5.91363106200984,-10.3565791710799));
#34355=CARTESIAN_POINT('Ctrl Pts',(219.559473917792,-4.20104299435734,-11.3344709853185));
#34356=CARTESIAN_POINT('Ctrl Pts',(219.598964968345,-2.24070553795645,-11.8784777420885));
#34357=CARTESIAN_POINT('Ctrl Pts',(219.638456018898,-0.269094468648538,
-11.9229758300881));
#34358=CARTESIAN_POINT('Ctrl Pts',(219.67794706945,1.70251660065938,-11.9674739180876));
#34359=CARTESIAN_POINT('Ctrl Pts',(219.717438120003,3.68540128287429,-11.5124633373165));
#34360=CARTESIAN_POINT('Ctrl Pts',(219.756929170556,5.44036392915078,-10.6128320802783));
#34361=CARTESIAN_POINT('Ctrl Pts',(219.796420221109,7.19532657542723,-9.71320082324006));
#34362=CARTESIAN_POINT('Ctrl Pts',(219.835911271661,8.72236718576524,-8.36894888993472));
#34363=CARTESIAN_POINT('Ctrl Pts',(219.875402322214,9.83727863996894,-6.74223356644574));
#34364=CARTESIAN_POINT('Ctrl Pts',(219.914893372767,10.9521900941726,-5.11551824295682));
#34365=CARTESIAN_POINT('Ctrl Pts',(219.95438442332,11.654972392242,-3.20633952928414));
#34366=CARTESIAN_POINT('Ctrl Pts',(219.993875473873,11.8608488152243,-1.24500193187064));
#34367=CARTESIAN_POINT('Ctrl Pts',(220.033366524425,12.0667252382066,0.716335665542974));
#34368=CARTESIAN_POINT('Ctrl Pts',(220.072857574978,11.7756957861018,2.72983214669756));
#34369=CARTESIAN_POINT('Ctrl Pts',(220.112348625531,11.0228673695967,4.55259919220793));
#34370=CARTESIAN_POINT('Ctrl Pts',(220.151839676084,10.2700389530916,6.3753662377182));
#34371=CARTESIAN_POINT('Ctrl Pts',(220.191330726636,9.05541157218612,8.00740384758426));
#34372=CARTESIAN_POINT('Ctrl Pts',(220.230821777189,7.52550591863462,9.25183902618784));
#34373=CARTESIAN_POINT('Ctrl Pts',(220.270312827742,5.99560026508303,10.4962742047915));
#34374=CARTESIAN_POINT('Ctrl Pts',(220.309803878295,4.15041633888536,11.3531069521326));
#34375=CARTESIAN_POINT('Ctrl Pts',(220.349294928847,2.21253887728794,11.7189775750894));
#34376=CARTESIAN_POINT('Ctrl Pts',(220.3887859794,0.274661415690581,12.0848481980461));
#34377=CARTESIAN_POINT('Ctrl Pts',(220.428277029953,-1.75590958130649,11.9597566966185));
#34378=CARTESIAN_POINT('Ctrl Pts',(220.467768080506,-3.63422594846958,11.3587925450367));
#34379=CARTESIAN_POINT('Ctrl Pts',(220.507259131059,-5.51254231563271,10.757828393455));
#34380=CARTESIAN_POINT('Ctrl Pts',(220.546750181611,-7.23860405296182,9.68099159171901));
#34381=CARTESIAN_POINT('Ctrl Pts',(220.586241232164,-8.60419632377035,8.25818180128231));
#34382=CARTESIAN_POINT('Ctrl Pts',(220.625732282717,-9.96978859457889,6.83537201084561));
#34383=CARTESIAN_POINT('Ctrl Pts',(220.66522333327,-10.9749113988668,5.06658923170817));
#34384=CARTESIAN_POINT('Ctrl Pts',(220.704714383822,-11.4983161621042,3.16520052856484));
#34385=CARTESIAN_POINT('Ctrl Pts',(220.726090640164,-11.7816318559873,2.13599082775773));
#34386=CARTESIAN_POINT('Ctrl Pts',(220.747466896506,-11.9238047153297,1.06792774302866));
#34387=CARTESIAN_POINT('Ctrl Pts',(220.768843152848,-11.9240373570162,-7.43698370121595E-5));
#34388=CARTESIAN_POINT('Origin',(201.227129595899,0.,0.));
#34389=CARTESIAN_POINT('',(219.977129595899,-11.0664557742297,-0.000226514961028955));
#34390=CARTESIAN_POINT('',(220.272870404101,-11.0650567036372,-6.90124023777772E-5));
#34391=CARTESIAN_POINT('',(201.227129595899,-11.06595,-5.55035408696717E-13));
#34392=CARTESIAN_POINT('',(221.275,-7.33091411968472,8.28932732930165));
#34393=CARTESIAN_POINT('Ctrl Pts',(219.977129595899,-11.0664557742297,-0.00022651496102942));
#34394=CARTESIAN_POINT('Ctrl Pts',(219.982711555224,-11.0666930110685,-0.258928326268467));
#34395=CARTESIAN_POINT('Ctrl Pts',(220.027784565101,-10.9949140254131,-2.34775325236548));
#34396=CARTESIAN_POINT('Ctrl Pts',(220.112348625531,-9.72987795281957,-6.18729765367837));
#34397=CARTESIAN_POINT('Ctrl Pts',(220.230821777189,-5.61014574409689,-10.0737005557397));
#34398=CARTESIAN_POINT('Ctrl Pts',(220.349294928847,-0.136908381828727,
-11.5297194437361));
#34399=CARTESIAN_POINT('Ctrl Pts',(220.467768080506,5.36935983023475,-10.20407562191));
#34400=CARTESIAN_POINT('Ctrl Pts',(220.586241232164,9.58021420357832,-6.41659256981546));
#34401=CARTESIAN_POINT('Ctrl Pts',(220.704714383822,11.4797447729354,-1.08104305857399));
#34402=CARTESIAN_POINT('Ctrl Pts',(220.823187535481,10.6096662804338,4.51532424750848));
#34403=CARTESIAN_POINT('Ctrl Pts',(220.941660687139,7.17990244444507,9.02231263897793));
#34404=CARTESIAN_POINT('Ctrl Pts',(221.060133838797,2.01790159414706,11.3525974650078));
#34405=CARTESIAN_POINT('Ctrl Pts',(221.171246943085,-3.27998607346621,10.9692951231732));
#34406=CARTESIAN_POINT('Ctrl Pts',(221.242868996819,-6.21473622449859,9.27482791577466));
#34407=CARTESIAN_POINT('Ctrl Pts',(221.275,-7.33129268303492,8.28936271098459));
#34408=CARTESIAN_POINT('',(221.275,5.44726799658334,9.63236838871412));
#34409=CARTESIAN_POINT('Origin',(221.275,0.,0.));
#34410=CARTESIAN_POINT('Ctrl Pts',(220.272870404101,-11.0650567036372,-6.90124023777772E-5));
#34411=CARTESIAN_POINT('Ctrl Pts',(220.290985198312,-11.0652396482432,-0.839923763907543));
#34412=CARTESIAN_POINT('Ctrl Pts',(220.348591043075,-10.7650251550423,-3.51056971559727));
#34413=CARTESIAN_POINT('Ctrl Pts',(220.445687938392,-8.639031892527,-7.6367698092379));
#34414=CARTESIAN_POINT('Ctrl Pts',(220.56416109005,-3.96073003010559,-10.828943343905));
#34415=CARTESIAN_POINT('Ctrl Pts',(220.682634241709,1.67312238226268,-11.4084734661502));
#34416=CARTESIAN_POINT('Ctrl Pts',(220.801107393367,6.9033507794017,-9.23569581394894));
#34417=CARTESIAN_POINT('Ctrl Pts',(220.919580545025,10.4680037040556,-4.83449558382035));
#34418=CARTESIAN_POINT('Ctrl Pts',(221.038053696683,11.5072892832615,0.732618747333446));
#34419=CARTESIAN_POINT('Ctrl Pts',(221.156526848342,9.7699936824466,6.12389733841086));
#34420=CARTESIAN_POINT('Ctrl Pts',(221.235508949447,7.04065173359568,8.73128281072966));
#34421=CARTESIAN_POINT('Ctrl Pts',(221.275,5.44726799658334,9.63236838871412));
#34422=CARTESIAN_POINT('Origin',(201.227129595899,0.,0.));
#34423=CARTESIAN_POINT('',(218.477129595899,-11.0661475744647,0.000270029283923045));
#34424=CARTESIAN_POINT('',(218.772870404101,-11.0665624442258,-0.000201279480846472));
#34425=CARTESIAN_POINT('',(201.227129595899,-11.06595,-5.55035408696717E-13));
#34426=CARTESIAN_POINT('Ctrl Pts',(218.477129595899,-11.0661475744646,0.000270029283922883));
#34427=CARTESIAN_POINT('Ctrl Pts',(218.50881894859,-11.064660089562,-1.46852466027703));
#34428=CARTESIAN_POINT('Ctrl Pts',(218.579999351834,-10.4036740682491,-4.7690199151945));
#34429=CARTESIAN_POINT('Ctrl Pts',(218.690670805631,-7.21724808383853,-8.99246948207381));
#34430=CARTESIAN_POINT('Ctrl Pts',(218.809143957289,-2.06496223864743,-11.3441221891729));
#34431=CARTESIAN_POINT('Ctrl Pts',(218.927617108948,3.58551696051438,-10.9588888768492));
#34432=CARTESIAN_POINT('Ctrl Pts',(219.046090260606,8.37095335800593,-7.92971103942582));
#34433=CARTESIAN_POINT('Ctrl Pts',(219.164563412264,11.1368112607131,-2.98740894949973));
#34434=CARTESIAN_POINT('Ctrl Pts',(219.283036563923,11.2157990354753,2.67563623960653));
#34435=CARTESIAN_POINT('Ctrl Pts',(219.401509715581,8.58886006959068,7.69315669910092));
#34436=CARTESIAN_POINT('Ctrl Pts',(219.519982867239,3.8897703770425,10.8546240695241));
#34437=CARTESIAN_POINT('Ctrl Pts',(219.638456018897,-1.74776638133898,11.3973018738637));
#34438=CARTESIAN_POINT('Ctrl Pts',(219.756929170556,-6.96363654138209,9.19026350689656));
#34439=CARTESIAN_POINT('Ctrl Pts',(219.86982036289,-10.3328647442766,4.97443341609356));
#34440=CARTESIAN_POINT('Ctrl Pts',(219.943220504671,-11.0650146161803,1.57132619810322));
#34441=CARTESIAN_POINT('Ctrl Pts',(219.977129595899,-11.0664557742297,-0.00022651496102942));
#34442=CARTESIAN_POINT('Ctrl Pts',(218.772870404101,-11.0665624442258,-0.000201279480847652));
#34443=CARTESIAN_POINT('Ctrl Pts',(218.777601541126,-11.0667474281854,-0.219464717225433));
#34444=CARTESIAN_POINT('Ctrl Pts',(218.821823728703,-11.007072604194,-2.26883103935306));
#34445=CARTESIAN_POINT('Ctrl Pts',(218.905536966834,-9.79547360465598,-6.08291662972795));
#34446=CARTESIAN_POINT('Ctrl Pts',(219.024010118492,-5.71752855338079,-10.0131436167636));
#34447=CARTESIAN_POINT('Ctrl Pts',(219.14248327015,-0.260170999755849,-11.5275968419408));
#34448=CARTESIAN_POINT('Ctrl Pts',(219.260956421809,5.25995547801919,-10.260898895706));
#34449=CARTESIAN_POINT('Ctrl Pts',(219.379429573467,9.51106366467834,-6.51865369284798));
#34450=CARTESIAN_POINT('Ctrl Pts',(219.497902725125,11.4675300222433,-1.2037162874228));
#34451=CARTESIAN_POINT('Ctrl Pts',(219.616375876784,10.657336974314,4.40162997311355));
#34452=CARTESIAN_POINT('Ctrl Pts',(219.734849028442,7.27595185085969,8.94503792000617));
#34453=CARTESIAN_POINT('Ctrl Pts',(219.8533221801,2.13916868907181,11.3303632886701));
#34454=CARTESIAN_POINT('Ctrl Pts',(219.971795331758,-3.51371109060621,10.9821227099977));
#34455=CARTESIAN_POINT('Ctrl Pts',(220.090268483417,-8.31887156411482,7.98433096001791));
#34456=CARTESIAN_POINT('Ctrl Pts',(220.190626840864,-10.6891769307306,3.81314382160942));
#34457=CARTESIAN_POINT('Ctrl Pts',(220.251494147759,-11.0648408209311,0.990996646370493));
#34458=CARTESIAN_POINT('Ctrl Pts',(220.272870404101,-11.0650567036372,-6.90124023777772E-5));
#34459=CARTESIAN_POINT('Origin',(201.227129595899,0.,0.));
#34460=CARTESIAN_POINT('',(216.977129595899,-11.0650512767152,-6.05169948032443E-5));
#34461=CARTESIAN_POINT('',(217.272870404101,-11.0660244859104,0.000277648619103621));
#34462=CARTESIAN_POINT('',(201.227129595899,-11.06595,-5.55035408696717E-13));
#34463=CARTESIAN_POINT('Ctrl Pts',(216.977129595899,-11.0650512767152,-6.05169948027923E-5));
#34464=CARTESIAN_POINT('Ctrl Pts',(216.995435291404,-11.0652148268645,-0.848767003760925));
#34465=CARTESIAN_POINT('Ctrl Pts',(217.053232037462,-10.7607722633556,-3.52828058602642));
#34466=CARTESIAN_POINT('Ctrl Pts',(217.150519834073,-8.62068509653071,-7.65747776726749));
#34467=CARTESIAN_POINT('Ctrl Pts',(217.268992985731,-3.93474448792423,-10.8384022394674));
#34468=CARTESIAN_POINT('Ctrl Pts',(217.38746613739,1.70049365109212,-11.4044508255478));
#34469=CARTESIAN_POINT('Ctrl Pts',(217.505939289048,6.92547022714963,-9.21905848894597));
#34470=CARTESIAN_POINT('Ctrl Pts',(217.624412440706,10.4796059636719,-4.80947358199571));
#34471=CARTESIAN_POINT('Ctrl Pts',(217.742885592365,11.5054291016218,0.760446235638654));
#34472=CARTESIAN_POINT('Ctrl Pts',(217.861358744023,9.75544927040927,6.14690058665455));
#34473=CARTESIAN_POINT('Ctrl Pts',(217.979831895681,5.65186708233216,10.0503520223619));
#34474=CARTESIAN_POINT('Ctrl Pts',(218.098305047339,0.184713897477963,11.5290527826799));
#34475=CARTESIAN_POINT('Ctrl Pts',(218.216778198998,-5.32700341275905,10.2262511180883));
#34476=CARTESIAN_POINT('Ctrl Pts',(218.335251350656,-9.55352642391547,6.4562613142035));
#34477=CARTESIAN_POINT('Ctrl Pts',(218.422035149623,-10.9611611781699,2.5536733215898));
#34478=CARTESIAN_POINT('Ctrl Pts',(218.469327898038,-11.0665137828848,0.361877049166292));
#34479=CARTESIAN_POINT('Ctrl Pts',(218.477129595899,-11.0661475744646,0.000270029283922883));
#34480=CARTESIAN_POINT('Ctrl Pts',(217.272870404101,-11.0660244859104,0.000277648619103552));
#34481=CARTESIAN_POINT('Ctrl Pts',(217.303708934492,-11.0645721443471,-1.42912743809139));
#34482=CARTESIAN_POINT('Ctrl Pts',(217.374038515437,-10.42991951896,-4.69024517517523));
#34483=CARTESIAN_POINT('Ctrl Pts',(217.483859146934,-7.31297897803034,-8.91479199580349));
#34484=CARTESIAN_POINT('Ctrl Pts',(217.602332298592,-2.18613040678854,-11.3213961906678));
#34485=CARTESIAN_POINT('Ctrl Pts',(217.720805450251,3.46814458380223,-10.9965972467579));
#34486=CARTESIAN_POINT('Ctrl Pts',(217.839278601909,8.28569406435969,-8.01875624603833));
#34487=CARTESIAN_POINT('Ctrl Pts',(217.957751753567,11.104234730707,-3.1063079221047));
#34488=CARTESIAN_POINT('Ctrl Pts',(218.076224905225,11.2437646914523,2.55556909998565));
#34489=CARTESIAN_POINT('Ctrl Pts',(218.194698056884,8.6706209101412,7.60088882263999));
#34490=CARTESIAN_POINT('Ctrl Pts',(218.313171208542,4.00560075861009,10.8124160308581));
#34491=CARTESIAN_POINT('Ctrl Pts',(218.4316443602,-1.62581172654604,11.4153367927059));
#34492=CARTESIAN_POINT('Ctrl Pts',(218.550117511859,-6.86498043029599,9.26419028054612));
#34493=CARTESIAN_POINT('Ctrl Pts',(218.663859526492,-10.3048207733217,5.05312341969914));
#34494=CARTESIAN_POINT('Ctrl Pts',(218.738110490573,-11.0652033573079,1.61073877485134));
#34495=CARTESIAN_POINT('Ctrl Pts',(218.772870404101,-11.0665624442258,-0.000201279480847652));
#34496=CARTESIAN_POINT('Origin',(201.227129595899,0.,0.));
#34497=CARTESIAN_POINT('',(215.477129595899,-11.0665392919594,-0.000207324146620239));
#34498=CARTESIAN_POINT('',(215.772870404101,-11.065081553347,-9.51519639225129E-5));
#34499=CARTESIAN_POINT('',(201.227129595899,-11.06595,-5.55035408696717E-13));
#34500=CARTESIAN_POINT('Ctrl Pts',(215.477129595899,-11.0665392919594,-0.000207324146620537));
#34501=CARTESIAN_POINT('Ctrl Pts',(215.482051634218,-11.0667359263627,-0.228319417445807));
#34502=CARTESIAN_POINT('Ctrl Pts',(215.52646472309,-11.0043819432692,-2.28653868628294));
#34503=CARTESIAN_POINT('Ctrl Pts',(215.610368862515,-9.7808528815819,-6.10639780874076));
#34504=CARTESIAN_POINT('Ctrl Pts',(215.728842014173,-5.6934912171844,-10.0268307580006));
#34505=CARTESIAN_POINT('Ctrl Pts',(215.847315165831,-0.232516305860531,
-11.5281877785388));
#34506=CARTESIAN_POINT('Ctrl Pts',(215.96578831749,5.28455555295532,-10.2482510653024));
#34507=CARTESIAN_POINT('Ctrl Pts',(216.084261469148,9.52667409494713,-6.4958184994969));
#34508=CARTESIAN_POINT('Ctrl Pts',(216.202734620806,11.4703846414241,-1.17620298738114));
#34509=CARTESIAN_POINT('Ctrl Pts',(216.321207772465,10.6467470547827,4.42718357889284));
#34510=CARTESIAN_POINT('Ctrl Pts',(216.439680924123,7.25447236425265,8.96246662510033));
#34511=CARTESIAN_POINT('Ctrl Pts',(216.558154075782,2.11198168868298,11.3354625241501));
#34512=CARTESIAN_POINT('Ctrl Pts',(216.67662722744,-3.54004626624265,10.9736616369653));
#34513=CARTESIAN_POINT('Ctrl Pts',(216.795100379098,-8.33800169158112,7.96435214445806));
#34514=CARTESIAN_POINT('Ctrl Pts',(216.895267835251,-10.6938035719187,3.79543445167127));
#34515=CARTESIAN_POINT('Ctrl Pts',(216.955944240852,-11.064861998576,0.982155550582976));
#34516=CARTESIAN_POINT('Ctrl Pts',(216.977129595899,-11.0650512767152,-6.05169948027923E-5));
#34517=CARTESIAN_POINT('Ctrl Pts',(215.772870404101,-11.065081553347,-9.51519639225129E-5));
#34518=CARTESIAN_POINT('Ctrl Pts',(215.790325277306,-11.0653275880705,-0.809348655494953));
#34519=CARTESIAN_POINT('Ctrl Pts',(215.847271201065,-10.7795512155158,-3.44933924082071));
#34520=CARTESIAN_POINT('Ctrl Pts',(215.943708175376,-8.70206265507251,-7.56487167166418));
#34521=CARTESIAN_POINT('Ctrl Pts',(216.062181327034,-4.05039886300789,-10.7957142844788));
#34522=CARTESIAN_POINT('Ctrl Pts',(216.180654478693,1.57846526560428,-11.4219799188598));
#34523=CARTESIAN_POINT('Ctrl Pts',(216.299127630351,6.8265084328873,-9.29257555671587));
#34524=CARTESIAN_POINT('Ctrl Pts',(216.417600782009,10.4275863101622,-4.92124187636331));
#34525=CARTESIAN_POINT('Ctrl Pts',(216.536073933668,11.512901864686,0.637391963915507));
#34526=CARTESIAN_POINT('Ctrl Pts',(216.654547085325,9.82061156918846,6.04224844479904));
#34527=CARTESIAN_POINT('Ctrl Pts',(216.773020236984,5.75899784281591,9.98935041471651));
#34528=CARTESIAN_POINT('Ctrl Pts',(216.891493388642,0.307966723115988,11.5264189737753));
#34529=CARTESIAN_POINT('Ctrl Pts',(217.009966540301,-5.21736453236138,10.2826205413801));
#34530=CARTESIAN_POINT('Ctrl Pts',(217.128439691959,-9.48395299500455,6.55803426722514));
#34531=CARTESIAN_POINT('Ctrl Pts',(217.216074313226,-10.9474406210577,2.63260814707565));
#34532=CARTESIAN_POINT('Ctrl Pts',(217.26421788394,-11.0664319766208,0.401332957488395));
#34533=CARTESIAN_POINT('Ctrl Pts',(217.272870404101,-11.0660244859104,0.000277648619103552));
#34534=CARTESIAN_POINT('Origin',(201.227129595899,0.,0.));
#34535=CARTESIAN_POINT('',(213.977129595899,-11.0660521098639,0.000276383857342581));
#34536=CARTESIAN_POINT('',(214.272870404101,-11.0666382248001,-0.000178769468103801));
#34537=CARTESIAN_POINT('',(201.227129595899,-11.06595,-5.55035408696717E-13));
#34538=CARTESIAN_POINT('Ctrl Pts',(213.977129595899,-11.0660521098639,0.000276383857342327));
#34539=CARTESIAN_POINT('Ctrl Pts',(214.008159027585,-11.0645897179147,-1.437966866595));
#34540=CARTESIAN_POINT('Ctrl Pts',(214.078679509824,-10.424073677229,-4.70792184462568));
#34541=CARTESIAN_POINT('Ctrl Pts',(214.188691042615,-7.2915719210082,-8.93230967950104));
#34542=CARTESIAN_POINT('Ctrl Pts',(214.307164194274,-2.15896482813512,-11.3266079724081));
#34543=CARTESIAN_POINT('Ctrl Pts',(214.425637345932,3.4945147091572,-10.9882457306536));
#34544=CARTESIAN_POINT('Ctrl Pts',(214.54411049759,8.30490667276723,-7.99885632114799));
#34545=CARTESIAN_POINT('Ctrl Pts',(214.662583649248,11.1116545830117,-3.0796606497433));
#34546=CARTESIAN_POINT('Ctrl Pts',(214.781056800907,11.2376016720611,2.58253479160174));
#34547=CARTESIAN_POINT('Ctrl Pts',(214.899529952565,8.65236191079344,7.62166718339193));
#34548=CARTESIAN_POINT('Ctrl Pts',(215.018003104223,3.9796509504845,10.8219940677331));
#34549=CARTESIAN_POINT('Ctrl Pts',(215.136476255882,-1.65319168566326,11.4114037059512));
#34550=CARTESIAN_POINT('Ctrl Pts',(215.25494940754,-6.88718484395786,9.24769496766087));
#34551=CARTESIAN_POINT('Ctrl Pts',(215.368500520879,-10.3111568532547,5.0354698445964));
#34552=CARTESIAN_POINT('Ctrl Pts',(215.442560583666,-11.0651582671375,1.60189514492085));
#34553=CARTESIAN_POINT('Ctrl Pts',(215.477129595899,-11.0665392919594,-0.000207324146620537));
#34554=CARTESIAN_POINT('Ctrl Pts',(214.272870404101,-11.0666382248001,-0.000178769468104391));
#34555=CARTESIAN_POINT('Ctrl Pts',(214.27694162012,-11.0667838005927,-0.188854579626239));
#34556=CARTESIAN_POINT('Ctrl Pts',(214.320503886693,-11.0162073889607,-2.20761953155798));
#34557=CARTESIAN_POINT('Ctrl Pts',(214.403557203818,-9.84558069118264,-6.00147637793954));
#34558=CARTESIAN_POINT('Ctrl Pts',(214.522030355476,-5.80036812003173,-9.96538546839381));
#34559=CARTESIAN_POINT('Ctrl Pts',(214.640503507134,-0.355757151167077,
-11.5250429374883));
#34560=CARTESIAN_POINT('Ctrl Pts',(214.758976658793,5.17468388520643,-10.3041653980194));
#34561=CARTESIAN_POINT('Ctrl Pts',(214.877449810451,9.4566792733418,-6.59730209879029));
#34562=CARTESIAN_POINT('Ctrl Pts',(214.995922962109,11.4571536357504,-1.29877189235286));
#34563=CARTESIAN_POINT('Ctrl Pts',(215.114396113768,10.6934719810851,4.31310037575084));
#34564=CARTESIAN_POINT('Ctrl Pts',(215.232869265426,7.34988035404288,8.88439286855379));
#34565=CARTESIAN_POINT('Ctrl Pts',(215.351342417084,2.23305458427189,11.3122343100387));
#34566=CARTESIAN_POINT('Ctrl Pts',(215.469815568742,-3.42251854473055,11.0108830105732));
#34567=CARTESIAN_POINT('Ctrl Pts',(215.588288720401,-8.25237391435474,8.05304306701711));
#34568=CARTESIAN_POINT('Ctrl Pts',(215.689306998854,-10.6730009525744,3.87435598552514));
#34569=CARTESIAN_POINT('Ctrl Pts',(215.750834226754,-11.0647709429668,1.02155957521071));
#34570=CARTESIAN_POINT('Ctrl Pts',(215.772870404101,-11.065081553347,-9.51519639225129E-5));
#34571=CARTESIAN_POINT('Origin',(201.227129595899,0.,0.));
#34572=CARTESIAN_POINT('',(212.477129595899,-11.0650735657267,-8.74940401521985E-5));
#34573=CARTESIAN_POINT('',(212.772870404101,-11.0659292686802,0.000280042182215501));
#34574=CARTESIAN_POINT('',(201.227129595899,-11.06595,-5.55035408696717E-13));
#34575=CARTESIAN_POINT('Ctrl Pts',(212.477129595899,-11.0650735657267,-8.74940401521251E-5));
#34576=CARTESIAN_POINT('Ctrl Pts',(212.494775370399,-11.06530206838,-0.818193363706625));
#34577=CARTESIAN_POINT('Ctrl Pts',(212.551912195452,-10.775377450498,-3.46705175012318));
#34578=CARTESIAN_POINT('Ctrl Pts',(212.648540071057,-8.68388996795875,-7.58572556280073));
#34579=CARTESIAN_POINT('Ctrl Pts',(212.767013222715,-4.02448899226784,-10.8053998371582));
#34580=CARTESIAN_POINT('Ctrl Pts',(212.885486374374,1.60586129747547,-11.4181603939958));
#34581=CARTESIAN_POINT('Ctrl Pts',(213.003959526032,6.84878105175381,-9.27617245392087));
#34582=CARTESIAN_POINT('Ctrl Pts',(213.12243267769,10.4393620179098,-4.89621261270018));
#34583=CARTESIAN_POINT('Ctrl Pts',(213.240905829349,11.5113396508456,0.665008821455645));
#34584=CARTESIAN_POINT('Ctrl Pts',(213.359378981007,9.806088333898,6.06579004561915));
#34585=CARTESIAN_POINT('Ctrl Pts',(213.477852132665,5.73501746579043,10.0031371057694));
#34586=CARTESIAN_POINT('Ctrl Pts',(213.596325284323,0.280314716669852,11.5271245742102));
#34587=CARTESIAN_POINT('Ctrl Pts',(213.714798435982,-5.24201683759653,10.2700748178432));
#34588=CARTESIAN_POINT('Ctrl Pts',(213.83327158764,-9.49965797713093,6.5352640044053));
#34589=CARTESIAN_POINT('Ctrl Pts',(213.920715307613,-10.9505570442949,2.61489706102027));
#34590=CARTESIAN_POINT('Ctrl Pts',(213.968667977032,-11.0664508990984,0.392480351575348));
#34591=CARTESIAN_POINT('Ctrl Pts',(213.977129595899,-11.0660521098639,0.000276383857342327));
#34592=CARTESIAN_POINT('Ctrl Pts',(212.772870404101,-11.0659292686802,0.000280042182215223));
#34593=CARTESIAN_POINT('Ctrl Pts',(212.803049013487,-11.0645204618591,-1.39857152109217));
#34594=CARTESIAN_POINT('Ctrl Pts',(212.872718673426,-10.4499369733853,-4.62913162145941));
#34595=CARTESIAN_POINT('Ctrl Pts',(212.981879383918,-7.3866553660777,-8.85384099497784));
#34596=CARTESIAN_POINT('Ctrl Pts',(213.100352535576,-2.27994036961207,-11.3028779420362));
#34597=CARTESIAN_POINT('Ctrl Pts',(213.218825687235,3.37683366346876,-11.0249794680452));
#34598=CARTESIAN_POINT('Ctrl Pts',(213.337298838893,8.21891188410895,-8.08719143478177));
#34599=CARTESIAN_POINT('Ctrl Pts',(213.455771990551,11.0780931775952,-3.1982853859645));
#34600=CARTESIAN_POINT('Ctrl Pts',(213.574245142209,11.2645706837284,2.46223986907059));
#34601=CARTESIAN_POINT('Ctrl Pts',(213.692718293868,8.73335478842003,7.52872446043392));
#34602=CARTESIAN_POINT('Ctrl Pts',(213.811191445526,4.09512733028103,10.7788269310876));
#34603=CARTESIAN_POINT('Ctrl Pts',(213.929664597184,-1.53109166664286,11.4284266708017));
#34604=CARTESIAN_POINT('Ctrl Pts',(214.048137748843,-6.78791906966887,9.32080106885565));
#34605=CARTESIAN_POINT('Ctrl Pts',(214.162539684481,-10.28272188813,5.11413873802353));
#34606=CARTESIAN_POINT('Ctrl Pts',(214.237450569567,-11.0653717062799,1.64131260416363));
#34607=CARTESIAN_POINT('Ctrl Pts',(214.272870404101,-11.0666382248001,-0.000178769468104391));
#34608=CARTESIAN_POINT('Origin',(201.227129595899,0.,0.));
#34609=CARTESIAN_POINT('',(210.977129595899,-11.0666169876618,-0.000185531372268859));
#34610=CARTESIAN_POINT('',(211.272870404101,-11.0651142296248,-0.000120992757266514));
#34611=CARTESIAN_POINT('',(201.227129595899,-11.06595,-5.55035408696717E-13));
#34612=CARTESIAN_POINT('Ctrl Pts',(210.977129595899,-11.0666169876618,-0.000185531372269392));
#34613=CARTESIAN_POINT('Ctrl Pts',(210.981391713213,-11.0667737867174,-0.197709538727662));
#34614=CARTESIAN_POINT('Ctrl Pts',(211.02514488108,-11.0135913758753,-2.22532648196755));
#34615=CARTESIAN_POINT('Ctrl Pts',(211.108389099499,-9.83115519349314,-6.02507799544502));
#34616=CARTESIAN_POINT('Ctrl Pts',(211.226862251157,-5.77644511420377,-9.97927147302517));
#34617=CARTESIAN_POINT('Ctrl Pts',(211.345335402816,-0.328108308124205,
-11.5258631879735));
#34618=CARTESIAN_POINT('Ctrl Pts',(211.463808554474,5.19938799803607,-10.2917220005022));
#34619=CARTESIAN_POINT('Ctrl Pts',(211.582281706132,9.47247853494596,-6.57459715075616));
#34620=CARTESIAN_POINT('Ctrl Pts',(211.700754857791,11.460236311957,-1.27128319576909));
#34621=CARTESIAN_POINT('Ctrl Pts',(211.819228009449,10.6830943445901,4.33874089043461));
#34622=CARTESIAN_POINT('Ctrl Pts',(211.937701161107,7.32854611626294,8.90199916375812));
#34623=CARTESIAN_POINT('Ctrl Pts',(212.056174312765,2.2059108492439,11.3175586861713));
#34624=CARTESIAN_POINT('Ctrl Pts',(212.174647464424,-3.44892307207615,11.0026409071933));
#34625=CARTESIAN_POINT('Ctrl Pts',(212.293120616082,-8.27166887053497,8.03322297623846));
#34626=CARTESIAN_POINT('Ctrl Pts',(212.393947993241,-10.6777090723953,3.85664871067693));
#34627=CARTESIAN_POINT('Ctrl Pts',(212.455284319846,-11.0647906819383,1.0127186349046));
#34628=CARTESIAN_POINT('Ctrl Pts',(212.477129595899,-11.0650735657267,-8.74940401521251E-5));
#34629=CARTESIAN_POINT('Ctrl Pts',(211.272870404101,-11.0651142296248,-0.000120992757266861));
#34630=CARTESIAN_POINT('Ctrl Pts',(211.289665356301,-11.0654163729725,-0.778772252662076));
#34631=CARTESIAN_POINT('Ctrl Pts',(211.345951359054,-10.7938026724476,-3.38810849938383));
#34632=CARTESIAN_POINT('Ctrl Pts',(211.44172841236,-8.7644967721873,-7.4924478104204));
#34633=CARTESIAN_POINT('Ctrl Pts',(211.560201564018,-4.13978539143139,-10.7617542610137));
#34634=CARTESIAN_POINT('Ctrl Pts',(211.678674715676,1.48369174414633,-11.4346769377148));
#34635=CARTESIAN_POINT('Ctrl Pts',(211.797147867335,6.74921300408072,-9.34886633165234));
#34636=CARTESIAN_POINT('Ctrl Pts',(211.915621018993,10.3864172902835,-5.00754567963735));
#34637=CARTESIAN_POINT('Ctrl Pts',(212.034094170651,11.5177917027214,0.541896811466134));
#34638=CARTESIAN_POINT('Ctrl Pts',(212.15256732231,9.87038054147729,5.96060112975038));
#34639=CARTESIAN_POINT('Ctrl Pts',(212.271040473968,5.84163867350336,9.94124919060903));
#34640=CARTESIAN_POINT('Ctrl Pts',(212.389513625626,0.403541462807075,11.523468755082));
#34641=CARTESIAN_POINT('Ctrl Pts',(212.507986777285,-5.13191427148244,10.325533098669));
#34642=CARTESIAN_POINT('Ctrl Pts',(212.626459928943,-9.42924296622852,6.636456505198));
#34643=CARTESIAN_POINT('Ctrl Pts',(212.714754471215,-10.9364980717932,2.6938341513483));
#34644=CARTESIAN_POINT('Ctrl Pts',(212.763557962934,-11.066363994829,0.431934222033988));
#34645=CARTESIAN_POINT('Ctrl Pts',(212.772870404101,-11.0659292686802,0.000280042182215223));
#34646=CARTESIAN_POINT('Origin',(201.227129595899,0.,0.));
#34647=CARTESIAN_POINT('',(209.477129595899,-11.0659567005612,0.00027966449786441));
#34648=CARTESIAN_POINT('',(209.772870404101,-11.0667065609126,-0.00015392667879921));
#34649=CARTESIAN_POINT('',(201.227129595899,-11.06595,-5.55035408696717E-13));
#34650=CARTESIAN_POINT('Ctrl Pts',(209.477129595899,-11.0659567005612,0.000279664497864693));
#34651=CARTESIAN_POINT('Ctrl Pts',(209.50749910658,-11.0645339567228,-1.40741057953197));
#34652=CARTESIAN_POINT('Ctrl Pts',(209.577359667813,-10.4441767046115,-4.64681166211135));
#34653=CARTESIAN_POINT('Ctrl Pts',(209.686711279599,-7.36539431433226,-8.87153559898989));
#34654=CARTESIAN_POINT('Ctrl Pts',(209.805184431257,-2.25281894488235,-11.3083148210209));
#34655=CARTESIAN_POINT('Ctrl Pts',(209.923657582916,3.40327213884093,-11.0168469190931));
#34656=CARTESIAN_POINT('Ctrl Pts',(210.042130734574,8.23828885633043,-8.06745151887539));
#34657=CARTESIAN_POINT('Ctrl Pts',(210.160603886232,11.0857337530526,-3.17170056060973));
#34658=CARTESIAN_POINT('Ctrl Pts',(210.279077037891,11.2586314950991,2.48925574164375));
#34659=CARTESIAN_POINT('Ctrl Pts',(210.397550189549,8.71526872597554,7.54965352342579));
#34660=CARTESIAN_POINT('Ctrl Pts',(210.516023341207,4.0692578423892,10.7886198330415));
#34661=CARTESIAN_POINT('Ctrl Pts',(210.634496492866,-1.55850330026388,11.4247207735161));
#34662=CARTESIAN_POINT('Ctrl Pts',(210.752969644524,-6.81025951080084,9.30449045812232));
#34663=CARTESIAN_POINT('Ctrl Pts',(210.867180678869,-10.2891458759462,5.09649002157397));
#34664=CARTESIAN_POINT('Ctrl Pts',(210.94190066266,-11.0653209502573,1.63246780871538));
#34665=CARTESIAN_POINT('Ctrl Pts',(210.977129595899,-11.0666169876618,-0.000185531372269392));
#34666=CARTESIAN_POINT('Ctrl Pts',(209.772870404101,-11.0667065609126,-0.000153926678798932));
#34667=CARTESIAN_POINT('Ctrl Pts',(209.776281699115,-11.0668149481323,-0.158243627877831));
#34668=CARTESIAN_POINT('Ctrl Pts',(209.819184044682,-11.0250845540694,-2.14641047456581));
#34669=CARTESIAN_POINT('Ctrl Pts',(209.901577440802,-9.89501069369702,-5.91962340298576));
#34670=CARTESIAN_POINT('Ctrl Pts',(210.02005059246,-5.88280879368037,-9.9169419963289));
#34671=CARTESIAN_POINT('Ctrl Pts',(210.138523744118,-0.451318836496845,
-11.5216964536208));
#34672=CARTESIAN_POINT('Ctrl Pts',(210.256996895777,5.08905642651245,-10.3467232759617));
#34673=CARTESIAN_POINT('Ctrl Pts',(210.375470047435,9.40164454536766,-6.67549681328017));
#34674=CARTESIAN_POINT('Ctrl Pts',(210.493943199093,11.4459893320066,-1.39373816520411));
#34675=CARTESIAN_POINT('Ctrl Pts',(210.612416350752,10.7288716045437,4.2242741334779));
#34676=CARTESIAN_POINT('Ctrl Pts',(210.73088950241,7.42330338187457,8.82313690034356));
#34677=CARTESIAN_POINT('Ctrl Pts',(210.849362654068,2.32678695671764,11.2933272475212));
#34678=CARTESIAN_POINT('Ctrl Pts',(210.967835805727,-3.33109072546143,11.0388863768181));
#34679=CARTESIAN_POINT('Ctrl Pts',(211.086308957385,-8.18530854892373,8.1212007622316));
#34680=CARTESIAN_POINT('Ctrl Pts',(211.187987156843,-10.6565440575799,3.9355649498659));
#34681=CARTESIAN_POINT('Ctrl Pts',(211.250174305748,-11.0647059238997,1.0521205001896));
#34682=CARTESIAN_POINT('Ctrl Pts',(211.272870404101,-11.0651142296248,-0.000120992757266861));
#34683=CARTESIAN_POINT('Origin',(201.227129595899,0.,0.));
#34684=CARTESIAN_POINT('',(207.977129595899,-11.0651039401686,-0.000113627027166958));
#34685=CARTESIAN_POINT('',(208.272870404101,-11.0658352981118,0.000279391217192781));
#34686=CARTESIAN_POINT('',(201.227129595899,-11.06595,-5.55035408696717E-13));
#34687=CARTESIAN_POINT('Ctrl Pts',(207.977129595899,-11.0651039401686,-0.000113627027167121));
#34688=CARTESIAN_POINT('Ctrl Pts',(207.994115449394,-11.0653905789061,-0.787617584544385));
#34689=CARTESIAN_POINT('Ctrl Pts',(208.050592353441,-10.7897081350621,-3.40582138748802));
#34690=CARTESIAN_POINT('Ctrl Pts',(208.146560308041,-8.74649764535955,-7.51345168544144));
#34691=CARTESIAN_POINT('Ctrl Pts',(208.265033459699,-4.11395673115298,-10.771654343876));
#34692=CARTESIAN_POINT('Ctrl Pts',(208.383506611358,1.51111850823841,-11.4310847317218));
#34693=CARTESIAN_POINT('Ctrl Pts',(208.501979763016,6.77162088338667,-9.33264849340337));
#34694=CARTESIAN_POINT('Ctrl Pts',(208.620452914674,10.3984001537186,-4.9826149292203));
#34695=CARTESIAN_POINT('Ctrl Pts',(208.738926066332,11.5164585613786,0.569525674392788));
#34696=CARTESIAN_POINT('Ctrl Pts',(208.857399217991,9.85605302940134,5.98426235816675));
#34697=CARTESIAN_POINT('Ctrl Pts',(208.975872369649,5.817773450173,9.95523427008149));
#34698=CARTESIAN_POINT('Ctrl Pts',(209.094345521308,0.375896258524645,11.5244036415153));
#34699=CARTESIAN_POINT('Ctrl Pts',(209.212818672966,-5.15666976717709,10.3131922411068));
#34700=CARTESIAN_POINT('Ctrl Pts',(209.331291824624,-9.44513623567911,6.61381726230806));
#34701=CARTESIAN_POINT('Ctrl Pts',(209.419395465602,-10.9396905378665,2.67612257791915));
#34702=CARTESIAN_POINT('Ctrl Pts',(209.468008056027,-11.0663840243592,0.423082087090511));
#34703=CARTESIAN_POINT('Ctrl Pts',(209.477129595899,-11.0659567005612,0.000279664497864693));
#34704=CARTESIAN_POINT('Ctrl Pts',(208.272870404101,-11.0658352981118,0.000279391217193198));
#34705=CARTESIAN_POINT('Ctrl Pts',(208.302389092482,-11.0644823738004,-1.36801666621322));
#34706=CARTESIAN_POINT('Ctrl Pts',(208.371398831416,-10.4696593756224,-4.56800686291313));
#34707=CARTESIAN_POINT('Ctrl Pts',(208.479899620902,-7.45982377135673,-8.79228111253593));
#34708=CARTESIAN_POINT('Ctrl Pts',(208.59837277256,-2.37359354017129,-11.2835823906954));
#34709=CARTESIAN_POINT('Ctrl Pts',(208.716845924218,3.28529051715118,-11.0526034977951));
#34710=CARTESIAN_POINT('Ctrl Pts',(208.835319075877,8.15156448652971,-8.15507046465587));
#34711=CARTESIAN_POINT('Ctrl Pts',(208.953792227535,11.0511897802984,-3.29004290266605));
#34712=CARTESIAN_POINT('Ctrl Pts',(209.072265379193,11.2846020076979,2.3687413090957));
#34713=CARTESIAN_POINT('Ctrl Pts',(209.190738530852,8.79548807096082,7.4560423453157));
#34714=CARTESIAN_POINT('Ctrl Pts',(209.30921168251,4.18437227866815,10.7444965677815));
#34715=CARTESIAN_POINT('Ctrl Pts',(209.427684834168,-1.43626631304541,11.4407306121404));
#34716=CARTESIAN_POINT('Ctrl Pts',(209.546157985827,-6.71039090158305,9.37677086258944));
#34717=CARTESIAN_POINT('Ctrl Pts',(209.661219842471,-10.2603183169951,5.17513671043559));
#34718=CARTESIAN_POINT('Ctrl Pts',(209.736790648562,-11.0655601973255,1.67189078030484));
#34719=CARTESIAN_POINT('Ctrl Pts',(209.772870404101,-11.0667065609126,-0.000153926678798932));
#34720=CARTESIAN_POINT('Origin',(201.227129595899,0.,0.));
#34721=CARTESIAN_POINT('',(206.477129595899,-11.0666876103725,-0.000161338566072536));
#34722=CARTESIAN_POINT('',(206.772870404101,-11.0651547064503,-0.000145660905285783));
#34723=CARTESIAN_POINT('',(201.227129595899,-11.06595,-5.55035408696717E-13));
#34724=CARTESIAN_POINT('Ctrl Pts',(206.477129595899,-11.0666876103725,-0.000161338566072901));
#34725=CARTESIAN_POINT('Ctrl Pts',(206.480731792208,-11.0668064580106,-0.167098809598976));
#34726=CARTESIAN_POINT('Ctrl Pts',(206.523825039069,-11.0225429972219,-2.16411670981007));
#34727=CARTESIAN_POINT('Ctrl Pts',(206.606409336483,-9.8807814135434,-5.94334383542404));
#34728=CARTESIAN_POINT('Ctrl Pts',(206.724882488141,-5.85900176316342,-9.93102591024465));
#34729=CARTESIAN_POINT('Ctrl Pts',(206.8433556398,-0.423677746264986,-11.5227459599084));
#34730=CARTESIAN_POINT('Ctrl Pts',(206.961828791458,5.11386287945728,-10.3344851705362));
#34731=CARTESIAN_POINT('Ctrl Pts',(207.080301943116,9.41763154941819,-6.65292366475841));
#34732=CARTESIAN_POINT('Ctrl Pts',(207.198775094774,11.4492998581925,-1.36627597758734));
#34733=CARTESIAN_POINT('Ctrl Pts',(207.317248246433,10.7187069544147,4.24999982531037));
#34734=CARTESIAN_POINT('Ctrl Pts',(207.435721398091,7.40211588169753,8.8409195089455));
#34735=CARTESIAN_POINT('Ctrl Pts',(207.554194549749,2.29968830857567,11.298876535884));
#34736=CARTESIAN_POINT('Ctrl Pts',(207.672667701408,-3.35756269431251,11.0308635221138));
#34737=CARTESIAN_POINT('Ctrl Pts',(207.791140853066,-8.20476720404479,8.10154136057916));
#34738=CARTESIAN_POINT('Ctrl Pts',(207.89262815123,-10.6613336413215,3.91785892862821));
#34739=CARTESIAN_POINT('Ctrl Pts',(207.954624398841,-11.0647241617092,1.04328002721838));
#34740=CARTESIAN_POINT('Ctrl Pts',(207.977129595899,-11.0651039401686,-0.000113627027167121));
#34741=CARTESIAN_POINT('Ctrl Pts',(206.772870404101,-11.0651547064503,-0.000145660905285783));
#34742=CARTESIAN_POINT('Ctrl Pts',(206.789005435296,-11.0655057942391,-0.748193683314034));
#34743=CARTESIAN_POINT('Ctrl Pts',(206.844631517043,-10.8077808658941,-3.32687665877076));
#34744=CARTESIAN_POINT('Ctrl Pts',(206.939748649344,-8.82632815191763,-7.41950869102601));
#34745=CARTESIAN_POINT('Ctrl Pts',(207.058221801002,-4.22888722542433,-10.7270541480969));
#34746=CARTESIAN_POINT('Ctrl Pts',(207.17669495266,1.3888161887093,-11.4465875899995));
#34747=CARTESIAN_POINT('Ctrl Pts',(207.295168104319,6.67145342963094,-9.40451418191398));
#34748=CARTESIAN_POINT('Ctrl Pts',(207.413641255977,10.3445339930023,-5.09350511231458));
#34749=CARTESIAN_POINT('Ctrl Pts',(207.532114407635,11.5218894583563,0.446364392591136));
#34750=CARTESIAN_POINT('Ctrl Pts',(207.650587559294,9.91947072438404,5.87854390216176));
#34751=CARTESIAN_POINT('Ctrl Pts',(207.769060710952,5.92387777273893,9.89246430345869));
#34752=CARTESIAN_POINT('Ctrl Pts',(207.88753386261,0.499088450816281,11.5197260635753));
#34753=CARTESIAN_POINT('Ctrl Pts',(208.006007014269,-5.04611108713692,10.3677355655817));
#34754=CARTESIAN_POINT('Ctrl Pts',(208.124480165927,-9.37388448524946,6.71442235183001));
#34755=CARTESIAN_POINT('Ctrl Pts',(208.213434629204,-10.9252921471334,2.75506174053056));
#34756=CARTESIAN_POINT('Ctrl Pts',(208.262898041929,-11.0662923594504,0.46253379991349));
#34757=CARTESIAN_POINT('Ctrl Pts',(208.272870404101,-11.0658352981118,0.000279391217193198));
#34758=CARTESIAN_POINT('Origin',(201.227129595899,0.,0.));
#34759=CARTESIAN_POINT('',(204.977129595899,-11.0658620952239,0.000280741946515456));
#34760=CARTESIAN_POINT('',(205.272870404101,-11.066766136903,-0.000127008754821079));
#34761=CARTESIAN_POINT('',(201.227129595899,-11.06595,-5.55035408696717E-13));
#34762=CARTESIAN_POINT('Ctrl Pts',(204.977129595899,-11.0658620952239,0.000280741946515339));
#34763=CARTESIAN_POINT('Ctrl Pts',(205.006839185574,-11.0644918505083,-1.37685467993411));
#34764=CARTESIAN_POINT('Ctrl Pts',(205.076039825802,-10.463984581982,-4.58569121052636));
#34765=CARTESIAN_POINT('Ctrl Pts',(205.184731516583,-7.43871005394589,-8.8101508004562));
#34766=CARTESIAN_POINT('Ctrl Pts',(205.303204668241,-2.34651819820973,-11.2892442895734));
#34767=CARTESIAN_POINT('Ctrl Pts',(205.4216778199,3.31179555484533,-11.0446903333316));
#34768=CARTESIAN_POINT('Ctrl Pts',(205.540150971558,8.17110447541142,-8.13549198319505));
#34769=CARTESIAN_POINT('Ctrl Pts',(205.658624123217,11.0590505604482,-3.26352232004452));
#34770=CARTESIAN_POINT('Ctrl Pts',(205.777097274875,11.2788870549277,2.39580548916746));
#34771=CARTESIAN_POINT('Ctrl Pts',(205.895570426533,8.777576190803,7.47712067870388));
#34772=CARTESIAN_POINT('Ctrl Pts',(206.014043578191,4.15858488930056,10.7545036577774));
#34773=CARTESIAN_POINT('Ctrl Pts',(206.13251672985,-1.46370773570288,11.4372521609064));
#34774=CARTESIAN_POINT('Ctrl Pts',(206.250989881508,-6.73286583398743,9.36064607483558));
#34775=CARTESIAN_POINT('Ctrl Pts',(206.365860836858,-10.2668305718026,5.15749310034477));
#34776=CARTESIAN_POINT('Ctrl Pts',(206.441240741655,-11.0655035256654,1.66304467597888));
#34777=CARTESIAN_POINT('Ctrl Pts',(206.477129595899,-11.0666876103725,-0.000161338566072901));
#34778=CARTESIAN_POINT('Ctrl Pts',(205.272870404101,-11.066766136903,-0.000127008754821131));
#34779=CARTESIAN_POINT('Ctrl Pts',(205.27562177811,-11.0668407583771,-0.127631986551504));
#34780=CARTESIAN_POINT('Ctrl Pts',(205.317864202671,-11.0337047479051,-2.08520391838922));
#34781=CARTESIAN_POINT('Ctrl Pts',(205.399597677786,-9.94376021587458,-5.83736334058754));
#34782=CARTESIAN_POINT('Ctrl Pts',(205.518070829444,-5.96484490322095,-9.86781652946403));
#34783=CARTESIAN_POINT('Ctrl Pts',(205.636543981102,-0.546849485135998,
-11.5175576204352));
#34784=CARTESIAN_POINT('Ctrl Pts',(205.755017132761,5.00307899201479,-10.3885696055));
#34785=CARTESIAN_POINT('Ctrl Pts',(205.873490284419,9.3459632629926,-6.75323245198365));
#34786=CARTESIAN_POINT('Ctrl Pts',(205.991963436077,11.4340378838074,-1.4886085900372));
#34787=CARTESIAN_POINT('Ctrl Pts',(206.110436587736,10.7635333998672,4.13515738637055));
#34788=CARTESIAN_POINT('Ctrl Pts',(206.228909739394,7.49621590665812,8.76127416208841));
#34789=CARTESIAN_POINT('Ctrl Pts',(206.347382891052,2.42035931523562,11.2736435390796));
#34790=CARTESIAN_POINT('Ctrl Pts',(206.46585604271,-3.23943382596151,11.0661305951517));
#34791=CARTESIAN_POINT('Ctrl Pts',(206.584329194369,-8.1176802770788,8.18879995973997));
#34792=CARTESIAN_POINT('Ctrl Pts',(206.686667314832,-10.639804868209,3.9967692784412));
#34793=CARTESIAN_POINT('Ctrl Pts',(206.749514384743,-11.0646464946538,1.08267989306887));
#34794=CARTESIAN_POINT('Ctrl Pts',(206.772870404101,-11.0651547064503,-0.000145660905285783));
#34795=CARTESIAN_POINT('Origin',(203.804782797639,0.,-4.68805434560642E-16));
#34796=CARTESIAN_POINT('',(204.,14.5,-1.77573785876366E-15));
#34797=CARTESIAN_POINT('Origin',(204.,0.,0.));
#34798=CARTESIAN_POINT('',(203.609565595278,15.3123475237772,1.87522173824257E-15));
#34799=CARTESIAN_POINT('',(203.804782797639,14.9061737618886,1.82547979850311E-15));
#34800=CARTESIAN_POINT('',(203.609565595278,-15.3123475237772,-1.87522173824257E-15));
#34801=CARTESIAN_POINT('Origin',(203.609565595278,0.,-9.37610869121283E-16));
#34802=CARTESIAN_POINT('Origin',(203.609565595278,0.,-9.37610869121283E-16));
#34803=CARTESIAN_POINT('Origin',(199.,0.,0.));
#34804=CARTESIAN_POINT('',(194.390434404722,-22.6876524762228,-2.77843609851737E-15));
#34805=CARTESIAN_POINT('',(199.,-19.,-2.32682891837997E-15));
#34806=CARTESIAN_POINT('',(194.390434404722,22.6876524762228,-2.77843609851737E-15));
#34807=CARTESIAN_POINT('Origin',(194.390434404722,0.,-1.38921804925869E-15));
#34808=CARTESIAN_POINT('Origin',(194.390434404722,0.,-1.38921804925869E-15));
#34809=CARTESIAN_POINT('Origin',(204.,12.,0.));
#34810=CARTESIAN_POINT('',(204.,6.4242839578383,-9.01020671414155));
#34811=CARTESIAN_POINT('Ctrl Pts',(204.,5.13002622089324,10.7654810839695));
#34812=CARTESIAN_POINT('Ctrl Pts',(204.,5.38136954563958,10.6351616725403));
#34813=CARTESIAN_POINT('Ctrl Pts',(204.,5.62773511945152,10.496037570914));
#34814=CARTESIAN_POINT('Ctrl Pts',(204.,5.86861265292755,10.3482717207313));
#34815=CARTESIAN_POINT('Ctrl Pts',(204.,5.94054489470907,10.3041450281793));
#34816=CARTESIAN_POINT('Ctrl Pts',(204.,6.01198756307411,10.2592473760111));
#34817=CARTESIAN_POINT('Ctrl Pts',(204.,6.08292661269302,10.2135823224016));
#34818=CARTESIAN_POINT('Ctrl Pts',(204.,6.32103183087106,10.0603086654917));
#34819=CARTESIAN_POINT('Ctrl Pts',(204.,6.55346587906383,9.89839258016546));
#34820=CARTESIAN_POINT('Ctrl Pts',(204.,6.77986031074224,9.72824991976574));
#34821=CARTESIAN_POINT('Ctrl Pts',(204.,6.94636210335151,9.60311849428924));
#34822=CARTESIAN_POINT('Ctrl Pts',(204.,7.1095965371914,9.47353648922993));
#34823=CARTESIAN_POINT('Ctrl Pts',(204.,7.26940436268983,9.3396565875382));
#34824=CARTESIAN_POINT('Ctrl Pts',(204.,7.35126323925222,9.27107885479835));
#34825=CARTESIAN_POINT('Ctrl Pts',(204.,7.43222284822467,9.20137326579582));
#34826=CARTESIAN_POINT('Ctrl Pts',(204.,7.51226055916463,9.13055939493385));
#34827=CARTESIAN_POINT('Ctrl Pts',(204.,7.55773359935015,9.09032683508698));
#34828=CARTESIAN_POINT('Ctrl Pts',(204.,7.60290904536994,9.04973652299996));
#34829=CARTESIAN_POINT('Ctrl Pts',(204.,7.6477826193096,9.00879196524232));
#34830=CARTESIAN_POINT('Ctrl Pts',(204.,7.67412699137662,8.98475423949447));
#34831=CARTESIAN_POINT('Ctrl Pts',(204.,7.70036463731238,8.96059682297449));
#34832=CARTESIAN_POINT('Ctrl Pts',(204.,7.72648757778976,8.93632726435297));
#34833=CARTESIAN_POINT('Ctrl Pts',(204.,7.93284762077082,8.74460814434789));
#34834=CARTESIAN_POINT('Ctrl Pts',(204.,8.13218640352905,8.54577234004366));
#34835=CARTESIAN_POINT('Ctrl Pts',(204.,8.32415293242165,8.34023927042099));
#34836=CARTESIAN_POINT('Ctrl Pts',(204.,8.51588514583175,8.13495707568082));
#34837=CARTESIAN_POINT('Ctrl Pts',(204.,8.70026349258579,7.92299346524614));
#34838=CARTESIAN_POINT('Ctrl Pts',(204.,8.87689960063644,7.70473209956972));
#34839=CARTESIAN_POINT('Ctrl Pts',(204.,9.05225022064303,7.48805915417246));
#34840=CARTESIAN_POINT('Ctrl Pts',(204.,9.21997123123925,7.2651792925663));
#34841=CARTESIAN_POINT('Ctrl Pts',(204.,9.3796390247399,7.03644147863572));
#34842=CARTESIAN_POINT('Ctrl Pts',(204.,9.43899734574093,6.95140559076701));
#34843=CARTESIAN_POINT('Ctrl Pts',(204.,9.49724219729021,6.86555986952368));
#34844=CARTESIAN_POINT('Ctrl Pts',(204.,9.55435010923125,6.77892151321272));
#34845=CARTESIAN_POINT('Ctrl Pts',(204.,9.58173223932997,6.73738011091989));
#34846=CARTESIAN_POINT('Ctrl Pts',(204.,9.60885297102288,6.69565647540693));
#34847=CARTESIAN_POINT('Ctrl Pts',(204.,9.63570963697724,6.65375247545265));
#34848=CARTESIAN_POINT('Ctrl Pts',(204.,9.65311703621794,6.62659200593547));
#34849=CARTESIAN_POINT('Ctrl Pts',(204.,9.67040803962745,6.59936427222682));
#34850=CARTESIAN_POINT('Ctrl Pts',(204.,9.68758144205299,6.57207101681937));
#34851=CARTESIAN_POINT('Ctrl Pts',(204.,9.80968961419899,6.37800757807052));
#34852=CARTESIAN_POINT('Ctrl Pts',(204.,9.92586564114257,6.18061434034615));
#34853=CARTESIAN_POINT('Ctrl Pts',(204.,10.0359210519606,5.98011103618573));
#34854=CARTESIAN_POINT('Ctrl Pts',(204.,10.169417593916,5.73690175136203));
#34855=CARTESIAN_POINT('Ctrl Pts',(204.,10.2939100827387,5.48911690808692));
#34856=CARTESIAN_POINT('Ctrl Pts',(204.,10.4093216513626,5.23730002890402));
#34857=CARTESIAN_POINT('Ctrl Pts',(204.,10.5254180230111,4.983988975761));
#34858=CARTESIAN_POINT('Ctrl Pts',(204.,10.6323255696679,4.72659728746502));
#34859=CARTESIAN_POINT('Ctrl Pts',(204.,10.729917585886,4.4656569428601));
#34860=CARTESIAN_POINT('Ctrl Pts',(204.,10.8274066332726,4.20499191506283));
#34861=CARTESIAN_POINT('Ctrl Pts',(204.,10.9155999298627,3.94078508903903));
#34862=CARTESIAN_POINT('Ctrl Pts',(204.,10.9943206955058,3.67355490271475));
#34863=CARTESIAN_POINT('Ctrl Pts',(204.,11.070722593291,3.41419648293933));
#34864=CARTESIAN_POINT('Ctrl Pts',(204.,11.1382016992343,3.15198962618184));
#34865=CARTESIAN_POINT('Ctrl Pts',(204.,11.1965490037965,2.88740594074757));
#34866=CARTESIAN_POINT('Ctrl Pts',(204.,11.2184292430073,2.78818705870972));
#34867=CARTESIAN_POINT('Ctrl Pts',(204.,11.239024842206,2.68863395369663));
#34868=CARTESIAN_POINT('Ctrl Pts',(204.,11.2583230272717,2.58877165055923));
#34869=CARTESIAN_POINT('Ctrl Pts',(204.,11.2646093596117,2.55624177152537));
#34870=CARTESIAN_POINT('Ctrl Pts',(204.,11.2707580139378,2.52367908422497));
#34871=CARTESIAN_POINT('Ctrl Pts',(204.,11.276768526349,2.49108445736322));
#34872=CARTESIAN_POINT('Ctrl Pts',(204.,11.2819534753436,2.46296680844873));
#34873=CARTESIAN_POINT('Ctrl Pts',(204.,11.2870354183249,2.43482633632079));
#34874=CARTESIAN_POINT('Ctrl Pts',(204.,11.2920119385415,2.40667621364387));
#34875=CARTESIAN_POINT('Ctrl Pts',(204.,11.3401602971382,2.13432080420421));
#34876=CARTESIAN_POINT('Ctrl Pts',(204.,11.3785026931062,1.86075051089294));
#34877=CARTESIAN_POINT('Ctrl Pts',(204.,11.4069431380994,1.58648424740416));
#34878=CARTESIAN_POINT('Ctrl Pts',(204.,11.4353262302546,1.31277106768745));
#34879=CARTESIAN_POINT('Ctrl Pts',(204.,11.4538473676115,1.03836410278021));
#34880=CARTESIAN_POINT('Ctrl Pts',(204.,11.4623602432515,0.763770255373622));
#34881=CARTESIAN_POINT('Ctrl Pts',(204.,11.4653760895116,0.666490221838948));
#34882=CARTESIAN_POINT('Ctrl Pts',(204.,11.4671353615187,0.569186696189433));
#34883=CARTESIAN_POINT('Ctrl Pts',(204.,11.4676299794862,0.471882172297525));
#34884=CARTESIAN_POINT('Ctrl Pts',(204.,11.4690308522032,0.196293209297684));
#34885=CARTESIAN_POINT('Ctrl Pts',(204.,11.4602910303519,-0.0793043509409153));
#34886=CARTESIAN_POINT('Ctrl Pts',(204.,11.4415458577,-0.354378400011464));
#34887=CARTESIAN_POINT('Ctrl Pts',(204.,11.4228350041333,-0.628948837304771));
#34888=CARTESIAN_POINT('Ctrl Pts',(204.,11.3941552173243,-0.902998297934441));
#34889=CARTESIAN_POINT('Ctrl Pts',(204.,11.355590982303,-1.17598467682026));
#34890=CARTESIAN_POINT('Ctrl Pts',(204.,11.3322925135319,-1.3409085919427));
#34891=CARTESIAN_POINT('Ctrl Pts',(204.,11.3053853286628,-1.50544419830023));
#34892=CARTESIAN_POINT('Ctrl Pts',(204.,11.2748795879635,-1.66946821774531));
#34893=CARTESIAN_POINT('Ctrl Pts',(204.,11.2605870333378,-1.74631677818365));
#34894=CARTESIAN_POINT('Ctrl Pts',(204.,11.2455044662696,-1.82305299259109));
#34895=CARTESIAN_POINT('Ctrl Pts',(204.,11.2296324649341,-1.89966391050251));
#34896=CARTESIAN_POINT('Ctrl Pts',(204.,11.2207832961272,-1.94237704608795));
#34897=CARTESIAN_POINT('Ctrl Pts',(204.,11.2116872345337,-1.98505777273071));
#34898=CARTESIAN_POINT('Ctrl Pts',(204.,11.2023523551507,-2.02766811322841));
#34899=CARTESIAN_POINT('Ctrl Pts',(204.,11.1437789246351,-2.29503459071588));
#34900=CARTESIAN_POINT('Ctrl Pts',(204.,11.0757667283023,-2.55984023401176));
#34901=CARTESIAN_POINT('Ctrl Pts',(204.,10.9984988879299,-2.82157931663494));
#34902=CARTESIAN_POINT('Ctrl Pts',(204.,10.9211642668246,-3.08354461404129));
#34903=CARTESIAN_POINT('Ctrl Pts',(204.,10.8345578076104,-3.34243866433772));
#34904=CARTESIAN_POINT('Ctrl Pts',(204.,10.738812096583,-3.59774315463838));
#34905=CARTESIAN_POINT('Ctrl Pts',(204.,10.6439399624884,-3.85071826526072));
#34906=CARTESIAN_POINT('Ctrl Pts',(204.,10.5400943383499,-4.10016957985931));
#34907=CARTESIAN_POINT('Ctrl Pts',(204.,10.4273575366565,-4.34557304492614));
#34908=CARTESIAN_POINT('Ctrl Pts',(204.,10.3326692805132,-4.55168875700633));
#34909=CARTESIAN_POINT('Ctrl Pts',(204.,10.2317079682769,-4.75494878389947));
#34910=CARTESIAN_POINT('Ctrl Pts',(204.,10.1244983728406,-4.95502732763819));
#34911=CARTESIAN_POINT('Ctrl Pts',(204.,10.015461477266,-5.15851604701587));
#34912=CARTESIAN_POINT('Ctrl Pts',(204.,9.89996122074432,-5.3587140873406));
#34913=CARTESIAN_POINT('Ctrl Pts',(204.,9.77819623555298,-5.55535964468922));
#34914=CARTESIAN_POINT('Ctrl Pts',(204.,9.72492405453176,-5.64139207602925));
#34915=CARTESIAN_POINT('Ctrl Pts',(204.,9.67045252598315,-5.72674429116772));
#34916=CARTESIAN_POINT('Ctrl Pts',(204.,9.61479723035913,-5.81139313701224));
#34917=CARTESIAN_POINT('Ctrl Pts',(204.,9.58095274764431,-5.86286885675988));
#34918=CARTESIAN_POINT('Ctrl Pts',(204.,9.54667050012853,-5.91408445789606));
#34919=CARTESIAN_POINT('Ctrl Pts',(204.,9.51195388615793,-5.96503458703567));
#34920=CARTESIAN_POINT('Ctrl Pts',(204.,9.49594011558806,-5.9885364089368));
#34921=CARTESIAN_POINT('Ctrl Pts',(204.,9.47983416005849,-6.01198133597758));
#34922=CARTESIAN_POINT('Ctrl Pts',(204.,9.46364417473069,-6.03535773337556));
#34923=CARTESIAN_POINT('Ctrl Pts',(204.,9.31055150742202,-6.25640518692579));
#34924=CARTESIAN_POINT('Ctrl Pts',(204.,9.14977308434649,-6.47158654910881));
#34925=CARTESIAN_POINT('Ctrl Pts',(204.,8.9817196830734,-6.68056443750362));
#34926=CARTESIAN_POINT('Ctrl Pts',(204.,8.81244499279347,-6.89106102409696));
#34927=CARTESIAN_POINT('Ctrl Pts',(204.,8.63578878909517,-7.0952641246414));
#34928=CARTESIAN_POINT('Ctrl Pts',(204.,8.45212755363202,-7.29279890909091));
#34929=CARTESIAN_POINT('Ctrl Pts',(204.,8.26882949894822,-7.48994307852151));
#34930=CARTESIAN_POINT('Ctrl Pts',(204.,8.07855362515398,-7.68044571246501));
#34931=CARTESIAN_POINT('Ctrl Pts',(204.,7.88163787795555,-7.86389759447329));
#34932=CARTESIAN_POINT('Ctrl Pts',(204.,7.6862339608845,-8.04594101582726));
#34933=CARTESIAN_POINT('Ctrl Pts',(204.,7.48429126870913,-8.22104191791924));
#34934=CARTESIAN_POINT('Ctrl Pts',(204.,7.27611121107159,-8.38875832568992));
#34935=CARTESIAN_POINT('Ctrl Pts',(204.,7.07157555393425,-8.5535386896949));
#34936=CARTESIAN_POINT('Ctrl Pts',(204.,6.86101854652668,-8.71119112116731));
#34937=CARTESIAN_POINT('Ctrl Pts',(204.,6.64470498300361,-8.86125088123046));
#34938=CARTESIAN_POINT('Ctrl Pts',(204.,6.57188067822712,-8.9117701252554));
#34939=CARTESIAN_POINT('Ctrl Pts',(204.,6.4984037733868,-8.96142840640969));
#34940=CARTESIAN_POINT('Ctrl Pts',(204.,6.42428395783811,-9.01020671414169));
#34941=CARTESIAN_POINT('',(204.,-6.42465676560637,-9.01028147758818));
#34942=CARTESIAN_POINT('Origin',(204.,0.,0.));
#34943=CARTESIAN_POINT('Ctrl Pts',(204.,-6.42465676560677,-9.01028147758789));
#34944=CARTESIAN_POINT('Ctrl Pts',(204.,-6.65054912801718,-8.86194699748741));
#34945=CARTESIAN_POINT('Ctrl Pts',(204.,-6.87070467837785,-8.70551035742835));
#34946=CARTESIAN_POINT('Ctrl Pts',(204.,-7.08464448205146,-8.54123692224679));
#34947=CARTESIAN_POINT('Ctrl Pts',(204.,-7.14173823356622,-8.49739755001365));
#34948=CARTESIAN_POINT('Ctrl Pts',(204.,-7.19838920257658,-8.45299978400815));
#34949=CARTESIAN_POINT('Ctrl Pts',(204.,-7.25458803292142,-8.40804809380943));
#34950=CARTESIAN_POINT('Ctrl Pts',(204.,-7.4639774887815,-8.24056400396366));
#34951=CARTESIAN_POINT('Ctrl Pts',(204.,-7.6670926166537,-8.06539371176003));
#34952=CARTESIAN_POINT('Ctrl Pts',(204.,-7.86365984101134,-7.88300433101605));
#34953=CARTESIAN_POINT('Ctrl Pts',(204.,-8.00894357130265,-7.74819950947673));
#34954=CARTESIAN_POINT('Ctrl Pts',(204.,-8.15064981364656,-7.6094500659697));
#34955=CARTESIAN_POINT('Ctrl Pts',(204.,-8.28865671380878,-7.46693033139527));
#34956=CARTESIAN_POINT('Ctrl Pts',(204.,-8.35438639477961,-7.39905128567645));
#34957=CARTESIAN_POINT('Ctrl Pts',(204.,-8.41927676170901,-7.33031681857506));
#34958=CARTESIAN_POINT('Ctrl Pts',(204.,-8.48331377713208,-7.26074491649885));
#34959=CARTESIAN_POINT('Ctrl Pts',(204.,-8.52430087856167,-7.21621519274132));
#34960=CARTESIAN_POINT('Ctrl Pts',(204.,-8.56493837736498,-7.17134238784771));
#34961=CARTESIAN_POINT('Ctrl Pts',(204.,-8.60522246310078,-7.12613111045349));
#34962=CARTESIAN_POINT('Ctrl Pts',(204.,-8.6307288154565,-7.09750504756524));
#34963=CARTESIAN_POINT('Ctrl Pts',(204.,-8.65608834062076,-7.06874902546348));
#34964=CARTESIAN_POINT('Ctrl Pts',(204.,-8.68129526525307,-7.03987015636087));
#34965=CARTESIAN_POINT('Ctrl Pts',(204.,-8.85913295253149,-6.83612648801025));
#34966=CARTESIAN_POINT('Ctrl Pts',(204.,-9.02945634830405,-6.62618328961249));
#34967=CARTESIAN_POINT('Ctrl Pts',(204.,-9.19199863370888,-6.41052061691195));
#34968=CARTESIAN_POINT('Ctrl Pts',(204.,-9.35567666968762,-6.1933510193907));
#34969=CARTESIAN_POINT('Ctrl Pts',(204.,-9.51146491604776,-5.97038128340569));
#34970=CARTESIAN_POINT('Ctrl Pts',(204.,-9.65905552542869,-5.74206275455145));
#34971=CARTESIAN_POINT('Ctrl Pts',(204.,-9.80619753499587,-5.51443819701386));
#34972=CARTESIAN_POINT('Ctrl Pts',(204.,-9.94519205346384,-5.28149679965102));
#34973=CARTESIAN_POINT('Ctrl Pts',(204.,-10.0756928459269,-5.04365469710717));
#34974=CARTESIAN_POINT('Ctrl Pts',(204.,-10.121650657997,-4.9598950321676));
#34975=CARTESIAN_POINT('Ctrl Pts',(204.,-10.1665546751333,-4.87552733484104));
#34976=CARTESIAN_POINT('Ctrl Pts',(204.,-10.2103884138121,-4.79056903948713));
#34977=CARTESIAN_POINT('Ctrl Pts',(204.,-10.2257962386725,-4.76070568366332));
#34978=CARTESIAN_POINT('Ctrl Pts',(204.,-10.2410718169294,-4.73076935251653));
#34979=CARTESIAN_POINT('Ctrl Pts',(204.,-10.2562144105126,-4.70076079351632));
#34980=CARTESIAN_POINT('Ctrl Pts',(204.,-10.2706014570784,-4.67224952605507));
#34981=CARTESIAN_POINT('Ctrl Pts',(204.,-10.284863946233,-4.6436819915071));
#34982=CARTESIAN_POINT('Ctrl Pts',(204.,-10.2990008454926,-4.61506022377236));
#34983=CARTESIAN_POINT('Ctrl Pts',(204.,-10.3969751316163,-4.41670008765512));
#34984=CARTESIAN_POINT('Ctrl Pts',(204.,-10.4889285784169,-4.21571654717207));
#34985=CARTESIAN_POINT('Ctrl Pts',(204.,-10.5747194144341,-4.01236004123072));
#34986=CARTESIAN_POINT('Ctrl Pts',(204.,-10.6797305993346,-3.76344408892707));
#34987=CARTESIAN_POINT('Ctrl Pts',(204.,-10.7755102375713,-3.51097344526088));
#34988=CARTESIAN_POINT('Ctrl Pts',(204.,-10.862082533099,-3.25549885901863));
#34989=CARTESIAN_POINT('Ctrl Pts',(204.,-10.9495611244006,-2.99734979664691));
#34990=CARTESIAN_POINT('Ctrl Pts',(204.,-11.0276387752821,-2.73613301072007));
#34991=CARTESIAN_POINT('Ctrl Pts',(204.,-11.0962936510127,-2.4723904858174));
#34992=CARTESIAN_POINT('Ctrl Pts',(204.,-11.1652522053208,-2.20748135833999));
#34993=CARTESIAN_POINT('Ctrl Pts',(204.,-11.224704598828,-1.9400234909498));
#34994=CARTESIAN_POINT('Ctrl Pts',(204.,-11.2745791857272,-1.67054859462426));
#34995=CARTESIAN_POINT('Ctrl Pts',(204.,-11.3233278278927,-1.40715723420891));
#34996=CARTESIAN_POINT('Ctrl Pts',(204.,-11.362926170186,-1.14183827806072));
#34997=CARTESIAN_POINT('Ctrl Pts',(204.,-11.3932597362624,-0.875080645215561));
#34998=CARTESIAN_POINT('Ctrl Pts',(204.,-11.4046348235411,-0.775046532898629));
#34999=CARTESIAN_POINT('Ctrl Pts',(204.,-11.4147065686262,-0.674810074975735));
#35000=CARTESIAN_POINT('Ctrl Pts',(204.,-11.4234671746766,-0.574397033518757));
#35001=CARTESIAN_POINT('Ctrl Pts',(204.,-11.4262148823748,-0.542903129396417));
#35002=CARTESIAN_POINT('Ctrl Pts',(204.,-11.4288336031237,-0.511391854752237));
#35003=CARTESIAN_POINT('Ctrl Pts',(204.,-11.4313230765255,-0.479864005876946));
#35004=CARTESIAN_POINT('Ctrl Pts',(204.,-11.4334153680567,-0.453366252918575));
#35005=CARTESIAN_POINT('Ctrl Pts',(204.,-11.4354160841983,-0.426860091688597));
#35006=CARTESIAN_POINT('Ctrl Pts',(204.,-11.4373246045135,-0.400354135471182));
#35007=CARTESIAN_POINT('Ctrl Pts',(204.,-11.4571851542671,-0.124526386594492));
#35008=CARTESIAN_POINT('Ctrl Pts',(204.,-11.467086561415,0.151537388123827));
#35009=CARTESIAN_POINT('Ctrl Pts',(204.,-11.4670322276902,0.427285070384512));
#35010=CARTESIAN_POINT('Ctrl Pts',(204.,-11.4669776265041,0.704390139058355));
#35011=CARTESIAN_POINT('Ctrl Pts',(204.,-11.4568691710756,0.98117661984866));
#35012=CARTESIAN_POINT('Ctrl Pts',(204.,-11.4366600361361,1.25709887328326));
#35013=CARTESIAN_POINT('Ctrl Pts',(204.,-11.4298934228941,1.34948576561938));
#35014=CARTESIAN_POINT('Ctrl Pts',(204.,-11.4219939898967,1.44177584848161));
#35015=CARTESIAN_POINT('Ctrl Pts',(204.,-11.412958684684,1.53394881608885));
#35016=CARTESIAN_POINT('Ctrl Pts',(204.,-11.3860912032069,1.80803535124878));
#35017=CARTESIAN_POINT('Ctrl Pts',(204.,-11.3491838657346,2.08108650375856));
#35018=CARTESIAN_POINT('Ctrl Pts',(204.,-11.3024701946929,2.35261240030303));
#35019=CARTESIAN_POINT('Ctrl Pts',(204.,-11.2555816827369,2.62515456970653));
#35020=CARTESIAN_POINT('Ctrl Pts',(204.,-11.1988131424943,2.89616064928337));
#35021=CARTESIAN_POINT('Ctrl Pts',(204.,-11.1323486392896,3.16512786231975));
#35022=CARTESIAN_POINT('Ctrl Pts',(204.,-11.0912368266875,3.33149831760495));
#35023=CARTESIAN_POINT('Ctrl Pts',(204.,-11.0464142478112,3.49708850676293));
#35024=CARTESIAN_POINT('Ctrl Pts',(204.,-10.997914928214,3.66177647998853));
#35025=CARTESIAN_POINT('Ctrl Pts',(204.,-10.9753867054638,3.73827502421373));
#35026=CARTESIAN_POINT('Ctrl Pts',(204.,-10.9520650672135,3.81457886186982));
#35027=CARTESIAN_POINT('Ctrl Pts',(204.,-10.9279529066472,3.89067554151667));
#35028=CARTESIAN_POINT('Ctrl Pts',(204.,-10.9143162205251,3.93371218820865));
#35029=CARTESIAN_POINT('Ctrl Pts',(204.,-10.9004243749725,3.97668935780195));
#35030=CARTESIAN_POINT('Ctrl Pts',(204.,-10.8862900827949,4.01956828440585));
#35031=CARTESIAN_POINT('Ctrl Pts',(204.,-10.798911086603,4.28464824153112));
#35032=CARTESIAN_POINT('Ctrl Pts',(204.,-10.702209612138,4.54617686608043));
#35033=CARTESIAN_POINT('Ctrl Pts',(204.,-10.5964725843817,4.80366716089838));
#35034=CARTESIAN_POINT('Ctrl Pts',(204.,-10.4901388166223,5.06261063406443));
#35035=CARTESIAN_POINT('Ctrl Pts',(204.,-10.3746670590857,5.31747067532474));
#35036=CARTESIAN_POINT('Ctrl Pts',(204.,-10.2502963436619,5.56774633407479));
#35037=CARTESIAN_POINT('Ctrl Pts',(204.,-10.1261430056542,5.8175845564411));
#35038=CARTESIAN_POINT('Ctrl Pts',(204.,-9.99312157354115,6.06285500942485));
#35039=CARTESIAN_POINT('Ctrl Pts',(204.,-9.85142032185599,6.30304466996495));
#35040=CARTESIAN_POINT('Ctrl Pts',(204.,-9.73102700503411,6.50711647282378));
#35041=CARTESIAN_POINT('Ctrl Pts',(204.,-9.60436711932939,6.70752057533099));
#35042=CARTESIAN_POINT('Ctrl Pts',(204.,-9.47152968713627,6.90392906505641));
#35043=CARTESIAN_POINT('Ctrl Pts',(204.,-9.33469133475788,7.10625316665515));
#35044=CARTESIAN_POINT('Ctrl Pts',(204.,-9.19129761317494,7.30433764131528));
#35045=CARTESIAN_POINT('Ctrl Pts',(204.,-9.04161060192979,7.49794996228298));
#35046=CARTESIAN_POINT('Ctrl Pts',(204.,-8.97612253451004,7.58265535270634));
#35047=CARTESIAN_POINT('Ctrl Pts',(204.,-8.90942958866847,7.66650449296753));
#35048=CARTESIAN_POINT('Ctrl Pts',(204.,-8.84155236887728,7.74947665964046));
#35049=CARTESIAN_POINT('Ctrl Pts',(204.,-8.79958392576119,7.80077829909983));
#35050=CARTESIAN_POINT('Ctrl Pts',(204.,-8.75716272620976,7.85174466108664));
#35051=CARTESIAN_POINT('Ctrl Pts',(204.,-8.71429349733821,7.90237068802365));
#35052=CARTESIAN_POINT('Ctrl Pts',(204.,-8.69465601284209,7.92556139719303));
#35053=CARTESIAN_POINT('Ctrl Pts',(204.,-8.67492989531673,7.94867431658233));
#35054=CARTESIAN_POINT('Ctrl Pts',(204.,-8.65511880737665,7.97170556570952));
#35055=CARTESIAN_POINT('Ctrl Pts',(204.,-8.47328695105665,8.18309298647266));
#35056=CARTESIAN_POINT('Ctrl Pts',(204.,-8.28422016552803,8.38769783304993));
#35057=CARTESIAN_POINT('Ctrl Pts',(204.,-8.08840339292777,8.58524924614487));
#35058=CARTESIAN_POINT('Ctrl Pts',(204.,-7.89034148593488,8.78506568212811));
#35059=CARTESIAN_POINT('Ctrl Pts',(204.,-7.68537355787534,8.97766647086422));
#35060=CARTESIAN_POINT('Ctrl Pts',(204.,-7.47395492068874,9.16274545557204));
#35061=CARTESIAN_POINT('Ctrl Pts',(204.,-7.26126910103603,9.34893375044942));
#35062=CARTESIAN_POINT('Ctrl Pts',(204.,-7.04205459398052,9.52751026475814));
#35063=CARTESIAN_POINT('Ctrl Pts',(204.,-6.81673413565081,9.69813036804369));
#35064=CARTESIAN_POINT('Ctrl Pts',(204.,-6.5921607892943,9.86818473343318));
#35065=CARTESIAN_POINT('Ctrl Pts',(204.,-6.36152144411965,10.0303357784069));
#35066=CARTESIAN_POINT('Ctrl Pts',(204.,-6.12520100238345,10.1842031840316));
#35067=CARTESIAN_POINT('Ctrl Pts',(204.,-5.8919943458718,10.3360432150853));
#35068=CARTESIAN_POINT('Ctrl Pts',(204.,-5.65325482885913,10.4798167914932));
#35069=CARTESIAN_POINT('Ctrl Pts',(204.,-5.40932671028307,10.6151148681509));
#35070=CARTESIAN_POINT('Ctrl Pts',(204.,-5.31683948747285,10.6664141748265));
#35071=CARTESIAN_POINT('Ctrl Pts',(204.,-5.22360612044888,10.7164945619684));
#35072=CARTESIAN_POINT('Ctrl Pts',(204.,-5.12964461189203,10.7653319110786));
#35073=CARTESIAN_POINT('Origin',(193.945217202361,0.,-6.94609024629344E-16));
#35074=CARTESIAN_POINT('',(193.5,23.,2.81668763803891E-15));
#35075=CARTESIAN_POINT('',(193.945217202361,22.8438262381114,2.79756186827814E-15));
#35076=CARTESIAN_POINT('',(193.5,-23.,-2.81668763803891E-15));
#35077=CARTESIAN_POINT('Origin',(193.5,0.,0.));
#35078=CARTESIAN_POINT('Origin',(193.5,0.,0.));
#35079=CARTESIAN_POINT('Origin',(172.4,0.,0.));
#35080=CARTESIAN_POINT('',(150.8,-23.,-2.81668763803891E-15));
#35081=CARTESIAN_POINT('',(172.4,-23.,-2.81668763803891E-15));
#35082=CARTESIAN_POINT('Origin',(150.8,0.,0.));
#35083=CARTESIAN_POINT('Origin',(221.275,1.39622887047493E-15,0.));
#35084=CARTESIAN_POINT('',(221.275,-3.97626028075622,-11.2425521648637));
#35085=CARTESIAN_POINT('Ctrl Pts',(221.275,-7.33129268303527,8.28936271098428));
#35086=CARTESIAN_POINT('Ctrl Pts',(221.275,-7.54044240726459,8.11822864204739));
#35087=CARTESIAN_POINT('Ctrl Pts',(221.275,-7.74303984010792,7.93963645727318));
#35088=CARTESIAN_POINT('Ctrl Pts',(221.275,-7.9386364087855,7.75390012992646));
#35089=CARTESIAN_POINT('Ctrl Pts',(221.275,-7.99083493314403,7.70433299143922));
#35090=CARTESIAN_POINT('Ctrl Pts',(221.275,-8.0425347325609,7.65425680143036));
#35091=CARTESIAN_POINT('Ctrl Pts',(221.275,-8.09372696932752,7.60367698297605));
#35092=CARTESIAN_POINT('Ctrl Pts',(221.275,-8.2844625113853,7.41522323101266));
#35093=CARTESIAN_POINT('Ctrl Pts',(221.275,-8.46815467022213,7.21978122775128));
#35094=CARTESIAN_POINT('Ctrl Pts',(221.275,-8.64458019562942,7.01784412483079));
#35095=CARTESIAN_POINT('Ctrl Pts',(221.275,-8.77497710607317,6.86859149109764));
#35096=CARTESIAN_POINT('Ctrl Pts',(221.275,-8.90140380117501,6.71578979350078));
#35097=CARTESIAN_POINT('Ctrl Pts',(221.275,-9.02375731675049,6.55962514529613));
#35098=CARTESIAN_POINT('Ctrl Pts',(221.275,-9.08203163297198,6.48524732256424));
#35099=CARTESIAN_POINT('Ctrl Pts',(221.275,-9.13938181707504,6.41010649667514));
#35100=CARTESIAN_POINT('Ctrl Pts',(221.275,-9.19579578858202,6.33422202283415));
#35101=CARTESIAN_POINT('Ctrl Pts',(221.275,-9.2319037344147,6.28565191869511));
#35102=CARTESIAN_POINT('Ctrl Pts',(221.275,-9.26762813104671,6.23677715628016));
#35103=CARTESIAN_POINT('Ctrl Pts',(221.275,-9.3029656706437,6.18760271728134));
#35104=CARTESIAN_POINT('Ctrl Pts',(221.275,-9.32534005840804,6.15646733041508));
#35105=CARTESIAN_POINT('Ctrl Pts',(221.275,-9.34755483887619,6.12521804388268));
#35106=CARTESIAN_POINT('Ctrl Pts',(221.275,-9.36960501376276,6.0938625344152));
#35107=CARTESIAN_POINT('Ctrl Pts',(221.275,-9.52517147372286,5.87264589403949));
#35108=CARTESIAN_POINT('Ctrl Pts',(221.275,-9.67261677905937,5.64604914273315));
#35109=CARTESIAN_POINT('Ctrl Pts',(221.275,-9.81172575201428,5.41457759690167));
#35110=CARTESIAN_POINT('Ctrl Pts',(221.275,-9.95180673910459,5.18148865997232));
#35111=CARTESIAN_POINT('Ctrl Pts',(221.275,-10.0834348779947,4.94345606619207));
#35112=CARTESIAN_POINT('Ctrl Pts',(221.275,-10.2063511861488,4.70096086776407));
#35113=CARTESIAN_POINT('Ctrl Pts',(221.275,-10.3288938920592,4.45920272979267));
#35114=CARTESIAN_POINT('Ctrl Pts',(221.275,-10.4427779783649,4.2130085234756));
#35115=CARTESIAN_POINT('Ctrl Pts',(221.275,-10.5477026047267,3.96282829554833));
#35116=CARTESIAN_POINT('Ctrl Pts',(221.275,-10.5846533860096,3.87472357500786));
#35117=CARTESIAN_POINT('Ctrl Pts',(221.275,-10.6204925884416,3.78612430462181));
#35118=CARTESIAN_POINT('Ctrl Pts',(221.275,-10.6552056411817,3.69704954625496));
#35119=CARTESIAN_POINT('Ctrl Pts',(221.275,-10.6674074915966,3.6657392237237));
#35120=CARTESIAN_POINT('Ctrl Pts',(221.275,-10.6794701918223,3.63437014916719));
#35121=CARTESIAN_POINT('Ctrl Pts',(221.275,-10.6913930859635,3.60294314311006));
#35122=CARTESIAN_POINT('Ctrl Pts',(221.275,-10.7027210784224,3.57308421092436));
#35123=CARTESIAN_POINT('Ctrl Pts',(221.275,-10.7139193143212,3.54318233971434));
#35124=CARTESIAN_POINT('Ctrl Pts',(221.275,-10.7249869794359,3.51323966015309));
#35125=CARTESIAN_POINT('Ctrl Pts',(221.275,-10.8016902710256,3.30572506176606));
#35126=CARTESIAN_POINT('Ctrl Pts',(221.275,-10.8721314855905,3.09623078013545));
#35127=CARTESIAN_POINT('Ctrl Pts',(221.275,-10.9361958062775,2.88502070154648));
#35128=CARTESIAN_POINT('Ctrl Pts',(221.275,-11.0146129270476,2.62649167848104));
#35129=CARTESIAN_POINT('Ctrl Pts',(221.275,-11.0834775056231,2.36539239768169));
#35130=CARTESIAN_POINT('Ctrl Pts',(221.275,-11.1428711824738,2.1022680602064));
#35131=CARTESIAN_POINT('Ctrl Pts',(221.275,-11.2028866308757,1.83638916641912));
#35132=CARTESIAN_POINT('Ctrl Pts',(221.275,-11.2532319736341,1.5684420208977));
#35133=CARTESIAN_POINT('Ctrl Pts',(221.275,-11.2939421486287,1.2989679208318));
#35134=CARTESIAN_POINT('Ctrl Pts',(221.275,-11.3348323955048,1.02830186548141));
#35135=CARTESIAN_POINT('Ctrl Pts',(221.275,-11.3660021414784,0.756094696820204));
#35136=CARTESIAN_POINT('Ctrl Pts',(221.275,-11.3874357123412,0.48288270138544));
#35137=CARTESIAN_POINT('Ctrl Pts',(221.275,-11.4083854089844,0.21583861151868));
#35138=CARTESIAN_POINT('Ctrl Pts',(221.275,-11.4200334438198,-0.0521660484121864));
#35139=CARTESIAN_POINT('Ctrl Pts',(221.275,-11.4223170737475,-0.320633072357773));
#35140=CARTESIAN_POINT('Ctrl Pts',(221.275,-11.4231734349703,-0.421308206337368));
#35141=CARTESIAN_POINT('Ctrl Pts',(221.275,-11.422712443048,-0.52204834128742));
#35142=CARTESIAN_POINT('Ctrl Pts',(221.275,-11.4209290367306,-0.622827041307124));
#35143=CARTESIAN_POINT('Ctrl Pts',(221.275,-11.4203696826865,-0.654435639336831));
#35144=CARTESIAN_POINT('Ctrl Pts',(221.275,-11.4196802325306,-0.686048029947425));
#35145=CARTESIAN_POINT('Ctrl Pts',(221.275,-11.4188605105267,-0.717663393991851));
#35146=CARTESIAN_POINT('Ctrl Pts',(221.275,-11.4181715705133,-0.744234706244506));
#35147=CARTESIAN_POINT('Ctrl Pts',(221.275,-11.4173906777833,-0.770804808474893));
#35148=CARTESIAN_POINT('Ctrl Pts',(221.275,-11.4165181156319,-0.797365069739118));
#35149=CARTESIAN_POINT('Ctrl Pts',(221.275,-11.4074380154237,-1.07375779827223));
#35150=CARTESIAN_POINT('Ctrl Pts',(221.275,-11.3884286589653,-1.34934424762446));
#35151=CARTESIAN_POINT('Ctrl Pts',(221.275,-11.3595511416112,-1.62357568033119));
#35152=CARTESIAN_POINT('Ctrl Pts',(221.275,-11.3305314725491,-1.89915703748129));
#35153=CARTESIAN_POINT('Ctrl Pts',(221.275,-11.2915463274116,-2.17337064059582));
#35154=CARTESIAN_POINT('Ctrl Pts',(221.275,-11.2426061724809,-2.44566894539353));
#35155=CARTESIAN_POINT('Ctrl Pts',(221.275,-11.2262195730029,-2.53684240542007));
#35156=CARTESIAN_POINT('Ctrl Pts',(221.275,-11.2087164795845,-2.62780117488787));
#35157=CARTESIAN_POINT('Ctrl Pts',(221.275,-11.1900959790274,-2.71852474022907));
#35158=CARTESIAN_POINT('Ctrl Pts',(221.275,-11.1347258388575,-2.98830140462323));
#35159=CARTESIAN_POINT('Ctrl Pts',(221.275,-11.0694790694482,-3.25599891097075));
#35160=CARTESIAN_POINT('Ctrl Pts',(221.275,-10.9946391192961,-3.52115447789874));
#35161=CARTESIAN_POINT('Ctrl Pts',(221.275,-10.9195190595718,-3.7873024641462));
#35162=CARTESIAN_POINT('Ctrl Pts',(221.275,-10.8347336613073,-4.05089003348519));
#35163=CARTESIAN_POINT('Ctrl Pts',(221.275,-10.7405185355667,-4.31143640220764));
#35164=CARTESIAN_POINT('Ctrl Pts',(221.275,-10.6822414940986,-4.47259812029723));
#35165=CARTESIAN_POINT('Ctrl Pts',(221.275,-10.6203555744656,-4.63259596628076));
#35166=CARTESIAN_POINT('Ctrl Pts',(221.275,-10.5549073629548,-4.79131221473031));
#35167=CARTESIAN_POINT('Ctrl Pts',(221.275,-10.5245062780325,-4.86503685954903));
#35168=CARTESIAN_POINT('Ctrl Pts',(221.275,-10.4933364763593,-4.93848492990648));
#35169=CARTESIAN_POINT('Ctrl Pts',(221.275,-10.4614021367911,-5.01164434495921));
#35170=CARTESIAN_POINT('Ctrl Pts',(221.275,-10.4433416048742,-5.05301980374264));
#35171=CARTESIAN_POINT('Ctrl Pts',(221.275,-10.4250335284866,-5.09430943985858));
#35172=CARTESIAN_POINT('Ctrl Pts',(221.275,-10.4064946029195,-5.13547602864041));
#35173=CARTESIAN_POINT('Ctrl Pts',(221.275,-10.2918858808873,-5.38997028795609));
#35174=CARTESIAN_POINT('Ctrl Pts',(221.275,-10.1683769645976,-5.63995820398864));
#35175=CARTESIAN_POINT('Ctrl Pts',(221.275,-10.0363041119217,-5.88498543783887));
#35176=CARTESIAN_POINT('Ctrl Pts',(221.275,-9.90348589380986,-6.13139550568774));
#35177=CARTESIAN_POINT('Ctrl Pts',(221.275,-9.76200657895998,-6.37278932900673));
#35178=CARTESIAN_POINT('Ctrl Pts',(221.275,-9.61215625301232,-6.60869368572787));
#35179=CARTESIAN_POINT('Ctrl Pts',(221.275,-9.46256785038424,-6.84418570532644));
#35180=CARTESIAN_POINT('Ctrl Pts',(221.275,-9.30463739618173,-7.07420800749294));
#35181=CARTESIAN_POINT('Ctrl Pts',(221.275,-9.13860575860143,-7.29827005837135));
#35182=CARTESIAN_POINT('Ctrl Pts',(221.275,-8.99754065062552,-7.48863942327735));
#35183=CARTESIAN_POINT('Ctrl Pts',(221.275,-8.85062667997815,-7.67470614113694));
#35184=CARTESIAN_POINT('Ctrl Pts',(221.275,-8.69798665733386,-7.85615340033203));
#35185=CARTESIAN_POINT('Ctrl Pts',(221.275,-8.54074929178595,-8.04306564344805));
#35186=CARTESIAN_POINT('Ctrl Pts',(221.275,-8.37743562834725,-8.22507625757405));
#35187=CARTESIAN_POINT('Ctrl Pts',(221.275,-8.20833061687298,-8.40198138569603));
#35188=CARTESIAN_POINT('Ctrl Pts',(221.275,-8.13434717435299,-8.4793773792494));
#35189=CARTESIAN_POINT('Ctrl Pts',(221.275,-8.05925495617845,-8.55579586853935));
#35190=CARTESIAN_POINT('Ctrl Pts',(221.275,-7.98307662016529,-8.6312183975156));
#35191=CARTESIAN_POINT('Ctrl Pts',(221.275,-7.93597560161412,-8.67785210103825));
#35192=CARTESIAN_POINT('Ctrl Pts',(221.275,-7.88845935284263,-8.72410503762538));
#35193=CARTESIAN_POINT('Ctrl Pts',(221.275,-7.84053310373852,-8.76997267154632));
#35194=CARTESIAN_POINT('Ctrl Pts',(221.275,-7.81857910575888,-8.79098366158319));
#35195=CARTESIAN_POINT('Ctrl Pts',(221.275,-7.7965450915264,-8.81190802326766));
#35196=CARTESIAN_POINT('Ctrl Pts',(221.275,-7.77443510921182,-8.83274228022652));
#35197=CARTESIAN_POINT('Ctrl Pts',(221.275,-7.571503372549,-9.02396504497532));
#35198=CARTESIAN_POINT('Ctrl Pts',(221.275,-7.36208531361138,-9.2076861345953));
#35199=CARTESIAN_POINT('Ctrl Pts',(221.275,-7.14669153075602,-9.3836868656952));
#35200=CARTESIAN_POINT('Ctrl Pts',(221.275,-6.9288281416759,-9.56170554037418));
#35201=CARTESIAN_POINT('Ctrl Pts',(221.275,-6.70485080477499,-9.73182622056391));
#35202=CARTESIAN_POINT('Ctrl Pts',(221.275,-6.47524434022513,-9.89379202155816));
#35203=CARTESIAN_POINT('Ctrl Pts',(221.275,-6.24426165088319,-10.0567286199175));
#35204=CARTESIAN_POINT('Ctrl Pts',(221.275,-6.00758168644788,-10.2114127023956));
#35205=CARTESIAN_POINT('Ctrl Pts',(221.275,-5.76566089151908,-10.3575457161937));
#35206=CARTESIAN_POINT('Ctrl Pts',(221.275,-5.52454223046687,-10.5031941985115));
#35207=CARTESIAN_POINT('Ctrl Pts',(221.275,-5.27821692212139,-10.6403485865904));
#35208=CARTESIAN_POINT('Ctrl Pts',(221.275,-5.02710751503102,-10.7686708798398));
#35209=CARTESIAN_POINT('Ctrl Pts',(221.275,-4.7793067248221,-10.8953023988939));
#35210=CARTESIAN_POINT('Ctrl Pts',(221.275,-4.52684655678323,-11.0133333108478));
#35211=CARTESIAN_POINT('Ctrl Pts',(221.275,-4.27011214160444,-11.1223927977311));
#35212=CARTESIAN_POINT('Ctrl Pts',(221.275,-4.17276935738525,-11.1637435223363));
#35213=CARTESIAN_POINT('Ctrl Pts',(221.275,-4.07481192872072,-11.2038040128707));
#35214=CARTESIAN_POINT('Ctrl Pts',(221.275,-3.97626028075543,-11.2425521648639));
#35215=CARTESIAN_POINT('',(221.275,-11.925,-1.46039130798322E-15));
#35216=CARTESIAN_POINT('Origin',(221.275,0.,0.));
#35217=CARTESIAN_POINT('',(221.275,6.22722261202592,-10.1702729013571));
#35218=CARTESIAN_POINT('Origin',(221.275,0.,0.));
#35219=CARTESIAN_POINT('Ctrl Pts',(221.275,6.22722261202635,-10.1702729013569));
#35220=CARTESIAN_POINT('Ctrl Pts',(221.275,6.46356696607157,-10.0143948603033));
#35221=CARTESIAN_POINT('Ctrl Pts',(221.275,6.6940404968013,-9.85028067913405));
#35222=CARTESIAN_POINT('Ctrl Pts',(221.275,6.91815274221079,-9.67814574681644));
#35223=CARTESIAN_POINT('Ctrl Pts',(221.275,6.98507843449569,-9.62674181977657));
#35224=CARTESIAN_POINT('Ctrl Pts',(221.275,7.05143664808183,-9.57462233097456));
#35225=CARTESIAN_POINT('Ctrl Pts',(221.275,7.11721378651107,-9.52179228723434));
#35226=CARTESIAN_POINT('Ctrl Pts',(221.275,7.33799317947798,-9.34446950813644));
#35227=CARTESIAN_POINT('Ctrl Pts',(221.275,7.55222908968855,-9.15914444417878));
#35228=CARTESIAN_POINT('Ctrl Pts',(221.275,7.75959855762187,-8.96626918346592));
#35229=CARTESIAN_POINT('Ctrl Pts',(221.275,7.91210843984702,-8.82441906643268));
#35230=CARTESIAN_POINT('Ctrl Pts',(221.275,8.06090364990992,-8.67848428279718));
#35231=CARTESIAN_POINT('Ctrl Pts',(221.275,8.20584177038155,-8.5286333250904));
#35232=CARTESIAN_POINT('Ctrl Pts',(221.275,8.28008388987517,-8.45187468718273));
#35233=CARTESIAN_POINT('Ctrl Pts',(221.275,8.35331377497516,-8.37408837062628));
#35234=CARTESIAN_POINT('Ctrl Pts',(221.275,8.42551096529891,-8.29529620810303));
#35235=CARTESIAN_POINT('Ctrl Pts',(221.275,8.46652945203915,-8.25053081959966));
#35236=CARTESIAN_POINT('Ctrl Pts',(221.275,8.50721457956437,-8.20544074571969));
#35237=CARTESIAN_POINT('Ctrl Pts',(221.275,8.54756245993294,-8.16002992098362));
#35238=CARTESIAN_POINT('Ctrl Pts',(221.275,8.57124988608984,-8.13337014238227));
#35239=CARTESIAN_POINT('Ctrl Pts',(221.275,8.59481865970039,-8.10660248462503));
#35240=CARTESIAN_POINT('Ctrl Pts',(221.275,8.61826163420111,-8.07973528909513));
#35241=CARTESIAN_POINT('Ctrl Pts',(221.275,8.80345110972847,-7.86749593146063));
#35242=CARTESIAN_POINT('Ctrl Pts',(221.275,8.98091389215197,-7.64891279700364));
#35243=CARTESIAN_POINT('Ctrl Pts',(221.275,9.15034475193748,-7.42443969561466));
#35244=CARTESIAN_POINT('Ctrl Pts',(221.275,9.31956880282469,-7.20024058820088));
#35245=CARTESIAN_POINT('Ctrl Pts',(221.275,9.48078087434829,-6.97016535470833));
#35246=CARTESIAN_POINT('Ctrl Pts',(221.275,9.63363482555217,-6.73463614949089));
#35247=CARTESIAN_POINT('Ctrl Pts',(221.275,9.7853763664071,-6.50082103228556));
#35248=CARTESIAN_POINT('Ctrl Pts',(221.275,9.92888129444408,-6.26163051176708));
#35249=CARTESIAN_POINT('Ctrl Pts',(221.275,10.0637647993104,-6.01745591892541));
#35250=CARTESIAN_POINT('Ctrl Pts',(221.275,10.1139092789555,-5.92668123218567));
#35251=CARTESIAN_POINT('Ctrl Pts',(221.275,10.1628617382439,-5.83521753754474));
#35252=CARTESIAN_POINT('Ctrl Pts',(221.275,10.2106006333088,-5.74308439237998));
#35253=CARTESIAN_POINT('Ctrl Pts',(221.275,10.2334904992998,-5.69890835220816));
#35254=CARTESIAN_POINT('Ctrl Pts',(221.275,10.2561013503811,-5.65457840069286));
#35255=CARTESIAN_POINT('Ctrl Pts',(221.275,10.2784307291743,-5.61009667518484));
#35256=CARTESIAN_POINT('Ctrl Pts',(221.275,10.2929037296767,-5.58126541921545));
#35257=CARTESIAN_POINT('Ctrl Pts',(221.275,10.3072539409162,-5.55237943416662));
#35258=CARTESIAN_POINT('Ctrl Pts',(221.275,10.3214803464741,-5.52344057897386));
#35259=CARTESIAN_POINT('Ctrl Pts',(221.275,10.4226344459013,-5.31767645791328));
#35260=CARTESIAN_POINT('Ctrl Pts',(221.275,10.5175408384123,-5.10922085610939));
#35261=CARTESIAN_POINT('Ctrl Pts',(221.275,10.606035053905,-4.89831200280797));
#35262=CARTESIAN_POINT('Ctrl Pts',(221.275,10.7133779963714,-4.64248085294634));
#35263=CARTESIAN_POINT('Ctrl Pts',(221.275,10.8112879352375,-4.38304038856547));
#35264=CARTESIAN_POINT('Ctrl Pts',(221.275,10.8997452377967,-4.12053919019108));
#35265=CARTESIAN_POINT('Ctrl Pts',(221.275,10.9887274077414,-3.85648042320802));
#35266=CARTESIAN_POINT('Ctrl Pts',(221.275,11.0681445478099,-3.58932386836834));
#35267=CARTESIAN_POINT('Ctrl Pts',(221.275,11.1379262532868,-3.31961183526273));
#35268=CARTESIAN_POINT('Ctrl Pts',(221.275,11.20763433117,-3.05018437886434));
#35269=CARTESIAN_POINT('Ctrl Pts',(221.275,11.2677273629663,-2.77820619727043));
#35270=CARTESIAN_POINT('Ctrl Pts',(221.275,11.3180837281662,-2.50421136753778));
#35271=CARTESIAN_POINT('Ctrl Pts',(221.275,11.3669567537033,-2.23828756113564));
#35272=CARTESIAN_POINT('Ctrl Pts',(221.275,11.4066581240996,-1.97046360811415));
#35273=CARTESIAN_POINT('Ctrl Pts',(221.275,11.4370292709931,-1.70123038134001));
#35274=CARTESIAN_POINT('Ctrl Pts',(221.275,11.4484184510781,-1.60026792129971));
#35275=CARTESIAN_POINT('Ctrl Pts',(221.275,11.4584950926119,-1.49910735081375));
#35276=CARTESIAN_POINT('Ctrl Pts',(221.275,11.4672491072449,-1.39777489293779));
#35277=CARTESIAN_POINT('Ctrl Pts',(221.275,11.4701007059261,-1.36476609464781));
#35278=CARTESIAN_POINT('Ctrl Pts',(221.275,11.4728119512237,-1.33173905908973));
#35279=CARTESIAN_POINT('Ctrl Pts',(221.275,11.4753824725815,-1.29869469870299));
#35280=CARTESIAN_POINT('Ctrl Pts',(221.275,11.4775999226471,-1.27018911212607));
#35281=CARTESIAN_POINT('Ctrl Pts',(221.275,11.4797125453341,-1.24167159445729));
#35282=CARTESIAN_POINT('Ctrl Pts',(221.275,11.4817193140495,-1.21315549880311));
#35283=CARTESIAN_POINT('Ctrl Pts',(221.275,11.5011350170463,-0.937259208618942));
#35284=CARTESIAN_POINT('Ctrl Pts',(221.275,11.5106714848227,-0.661179693776942));
#35285=CARTESIAN_POINT('Ctrl Pts',(221.275,11.5102874958201,-0.385443059455608));
#35286=CARTESIAN_POINT('Ctrl Pts',(221.275,11.5099042811777,-0.110262481327592));
#35287=CARTESIAN_POINT('Ctrl Pts',(221.275,11.4996406157499,0.164577224029352));
#35288=CARTESIAN_POINT('Ctrl Pts',(221.275,11.4794039795718,0.438556636957472));
#35289=CARTESIAN_POINT('Ctrl Pts',(221.275,11.4722347702517,0.535619001641185));
#35290=CARTESIAN_POINT('Ctrl Pts',(221.275,11.4638134144713,0.63257338158797));
#35291=CARTESIAN_POINT('Ctrl Pts',(221.275,11.4541342279419,0.729396561550147));
#35292=CARTESIAN_POINT('Ctrl Pts',(221.275,11.4267205290986,1.00362224037745));
#35293=CARTESIAN_POINT('Ctrl Pts',(221.275,11.3892207871223,1.27679647484803));
#35294=CARTESIAN_POINT('Ctrl Pts',(221.275,11.3418252254633,1.54840422003022));
#35295=CARTESIAN_POINT('Ctrl Pts',(221.275,11.2945164335928,1.81951471724761));
#35296=CARTESIAN_POINT('Ctrl Pts',(221.275,11.2373477738928,2.08906505227169));
#35297=CARTESIAN_POINT('Ctrl Pts',(221.275,11.1704599346459,2.35652492196683));
#35298=CARTESIAN_POINT('Ctrl Pts',(221.275,11.1300498473678,2.51810999930639));
#35299=CARTESIAN_POINT('Ctrl Pts',(221.275,11.0860914022179,2.67893168126456));
#35300=CARTESIAN_POINT('Ctrl Pts',(221.275,11.0386075900197,2.83886842734617));
#35301=CARTESIAN_POINT('Ctrl Pts',(221.275,11.0163604629247,2.91380203003167));
#35302=CARTESIAN_POINT('Ctrl Pts',(221.275,10.9933393942903,2.98854132328388));
#35303=CARTESIAN_POINT('Ctrl Pts',(221.275,10.969546312832,3.06307348804126));
#35304=CARTESIAN_POINT('Ctrl Pts',(221.275,10.9562808923639,3.1046276055958));
#35305=CARTESIAN_POINT('Ctrl Pts',(221.275,10.9427733197184,3.14612368453342));
#35306=CARTESIAN_POINT('Ctrl Pts',(221.275,10.9290355953377,3.18752479983685));
#35307=CARTESIAN_POINT('Ctrl Pts',(221.275,10.8428356196636,3.44730400585014));
#35308=CARTESIAN_POINT('Ctrl Pts',(221.275,10.747516265156,3.70354978717551));
#35309=CARTESIAN_POINT('Ctrl Pts',(221.275,10.6433125138665,3.95577833042948));
#35310=CARTESIAN_POINT('Ctrl Pts',(221.275,10.5390186962296,4.20822488218407));
#35311=CARTESIAN_POINT('Ctrl Pts',(221.275,10.4258248653737,4.45664784193506));
#35312=CARTESIAN_POINT('Ctrl Pts',(221.275,10.3039170603746,4.70054559637153));
#35313=CARTESIAN_POINT('Ctrl Pts',(221.275,10.1831215214782,4.94221806913078));
#35314=CARTESIAN_POINT('Ctrl Pts',(221.275,10.0537699862449,5.17944806618623));
#35315=CARTESIAN_POINT('Ctrl Pts',(221.275,9.91599909542756,5.41172300983443));
#35316=CARTESIAN_POINT('Ctrl Pts',(221.275,9.80028461062045,5.60681193811528));
#35317=CARTESIAN_POINT('Ctrl Pts',(221.275,9.67862993840671,5.79840511634343));
#35318=CARTESIAN_POINT('Ctrl Pts',(221.275,9.55109377146823,5.98618112170417));
#35319=CARTESIAN_POINT('Ctrl Pts',(221.275,9.42138382955108,6.17715765278124));
#35320=CARTESIAN_POINT('Ctrl Pts',(221.275,9.28558990525997,6.36418593019245));
#35321=CARTESIAN_POINT('Ctrl Pts',(221.275,9.14393690820591,6.54702634593604));
#35322=CARTESIAN_POINT('Ctrl Pts',(221.275,9.08196372199475,6.62701902782386));
#35323=CARTESIAN_POINT('Ctrl Pts',(221.275,9.01886886064511,6.70620985440605));
#35324=CARTESIAN_POINT('Ctrl Pts',(221.275,8.95467023937287,6.7845774279421));
#35325=CARTESIAN_POINT('Ctrl Pts',(221.275,8.91563048444777,6.83223344927547));
#35326=CARTESIAN_POINT('Ctrl Pts',(221.275,8.87618255274118,6.87958501825374));
#35327=CARTESIAN_POINT('Ctrl Pts',(221.275,8.836330383554,6.92662716602368));
#35328=CARTESIAN_POINT('Ctrl Pts',(221.275,8.81794772954525,6.94832634937858));
#35329=CARTESIAN_POINT('Ctrl Pts',(221.275,8.79947934272416,6.96995931363031));
#35330=CARTESIAN_POINT('Ctrl Pts',(221.275,8.78093454974258,6.99151534017595));
#35331=CARTESIAN_POINT('Ctrl Pts',(221.275,8.60557477544427,7.1953493734579));
#35332=CARTESIAN_POINT('Ctrl Pts',(221.275,8.4231845219114,7.39254607125566));
#35333=CARTESIAN_POINT('Ctrl Pts',(221.275,8.2342075818506,7.5828128355903));
#35334=CARTESIAN_POINT('Ctrl Pts',(221.275,8.04385731241664,7.77446230268281));
#35335=CARTESIAN_POINT('Ctrl Pts',(221.275,7.84682381483834,7.9590811824017));
#35336=CARTESIAN_POINT('Ctrl Pts',(221.275,7.64352068799585,8.13633604943754));
#35337=CARTESIAN_POINT('Ctrl Pts',(221.275,7.44061961337772,8.31324037728258));
#35338=CARTESIAN_POINT('Ctrl Pts',(221.275,7.23147317562663,8.48281017305945));
#35339=CARTESIAN_POINT('Ctrl Pts',(221.275,7.01646024296744,8.64467378549681));
#35340=CARTESIAN_POINT('Ctrl Pts',(221.275,6.80309809964125,8.80529466931544));
#35341=CARTESIAN_POINT('Ctrl Pts',(221.275,6.58395869341164,8.95832757843745));
#35342=CARTESIAN_POINT('Ctrl Pts',(221.275,6.35938798073357,9.10336446350721));
#35343=CARTESIAN_POINT('Ctrl Pts',(221.275,6.13874862336006,9.24586231968636));
#35344=CARTESIAN_POINT('Ctrl Pts',(221.275,5.91286597430829,9.38064188928147));
#35345=CARTESIAN_POINT('Ctrl Pts',(221.275,5.68205195455429,9.50726865664796));
#35346=CARTESIAN_POINT('Ctrl Pts',(221.275,5.60434579241614,9.54989899654888));
#35347=CARTESIAN_POINT('Ctrl Pts',(221.275,5.52608059861463,9.59160487181287));
#35348=CARTESIAN_POINT('Ctrl Pts',(221.275,5.44726799658347,9.63236838871404));
#35349=CARTESIAN_POINT('Ctrl Pts',(203.504027251253,-4.76011662834041,9.98982177454118));
#35350=CARTESIAN_POINT('Ctrl Pts',(203.543518301805,-6.41263020639832,9.20240458742794));
#35351=CARTESIAN_POINT('Ctrl Pts',(203.622500402911,-9.31767905895346,6.7923303895484));
#35352=CARTESIAN_POINT('Ctrl Pts',(203.740973554569,-11.4278517756257,1.53578666224697));
#35353=CARTESIAN_POINT('Ctrl Pts',(203.859446706228,-10.780545153515,-4.09039060373519));
#35354=CARTESIAN_POINT('Ctrl Pts',(203.977919857886,-7.53249900452806,-8.73016539923752));
#35355=CARTESIAN_POINT('Ctrl Pts',(204.096393009544,-2.46707396923755,-11.263487531142));
#35356=CARTESIAN_POINT('Ctrl Pts',(204.214866161202,3.19351689060185,-11.0794786062488));
#35357=CARTESIAN_POINT('Ctrl Pts',(204.333339312861,8.08365868074054,-8.22238332192522));
#35358=CARTESIAN_POINT('Ctrl Pts',(204.451812464519,11.0235253467705,-3.38157672049597));
#35359=CARTESIAN_POINT('Ctrl Pts',(204.570285616177,11.303857784602,2.27508107448027));
#35360=CARTESIAN_POINT('Ctrl Pts',(204.688758767836,8.85701624610765,7.38284688961676));
#35361=CARTESIAN_POINT('Ctrl Pts',(204.807231919494,4.27332958062524,10.7094275823243));
#35362=CARTESIAN_POINT('Ctrl Pts',(204.925705071152,-1.34134224161475,11.4522476363554));
#35363=CARTESIAN_POINT('Ctrl Pts',(205.044178222811,-6.63240123149158,9.43209587689214));
#35364=CARTESIAN_POINT('Ctrl Pts',(205.162651374469,-10.3233254010507,5.13635381066313));
#35365=CARTESIAN_POINT('Ctrl Pts',(205.281124526127,-11.5236412090866,-0.398586246501114));
#35366=CARTESIAN_POINT('Ctrl Pts',(205.399597677786,-9.94376021587458,-5.83736334058754));
#35367=CARTESIAN_POINT('Ctrl Pts',(205.518070829444,-5.96484490322095,-9.86781652946403));
#35368=CARTESIAN_POINT('Ctrl Pts',(205.636543981102,-0.546849485135998,
-11.5175576204352));
#35369=CARTESIAN_POINT('Ctrl Pts',(205.755017132761,5.00307899201479,-10.3885696055));
#35370=CARTESIAN_POINT('Ctrl Pts',(205.873490284419,9.3459632629926,-6.75323245198365));
#35371=CARTESIAN_POINT('Ctrl Pts',(205.991963436077,11.4340378838074,-1.4886085900372));
#35372=CARTESIAN_POINT('Ctrl Pts',(206.110436587736,10.7635333998672,4.13515738637055));
#35373=CARTESIAN_POINT('Ctrl Pts',(206.228909739394,7.49621590665812,8.76127416208841));
#35374=CARTESIAN_POINT('Ctrl Pts',(206.347382891052,2.42035931523562,11.2736435390796));
#35375=CARTESIAN_POINT('Ctrl Pts',(206.46585604271,-3.23943382596151,11.0661305951517));
#35376=CARTESIAN_POINT('Ctrl Pts',(206.584329194369,-8.1176802770788,8.18879995973997));
#35377=CARTESIAN_POINT('Ctrl Pts',(206.702802346027,-11.0374529662102,3.33583720829552));
#35378=CARTESIAN_POINT('Ctrl Pts',(206.821275497686,-11.2943267364968,-2.32193053962052));
#35379=CARTESIAN_POINT('Ctrl Pts',(206.939748649344,-8.82632815191763,-7.41950869102601));
#35380=CARTESIAN_POINT('Ctrl Pts',(207.058221801002,-4.22888722542433,-10.7270541480969));
#35381=CARTESIAN_POINT('Ctrl Pts',(207.17669495266,1.3888161887093,-11.4465875899995));
#35382=CARTESIAN_POINT('Ctrl Pts',(207.295168104319,6.67145342963094,-9.40451418191398));
#35383=CARTESIAN_POINT('Ctrl Pts',(207.413641255977,10.3445339930023,-5.09350511231458));
#35384=CARTESIAN_POINT('Ctrl Pts',(207.532114407635,11.5218894583563,0.446364392591136));
#35385=CARTESIAN_POINT('Ctrl Pts',(207.650587559294,9.91947072438404,5.87854390216176));
#35386=CARTESIAN_POINT('Ctrl Pts',(207.769060710952,5.92387777273893,9.89246430345869));
#35387=CARTESIAN_POINT('Ctrl Pts',(207.88753386261,0.499088450816281,11.5197260635753));
#35388=CARTESIAN_POINT('Ctrl Pts',(208.006007014269,-5.04611108713692,10.3677355655817));
#35389=CARTESIAN_POINT('Ctrl Pts',(208.124480165927,-9.37388448524946,6.71442235183001));
#35390=CARTESIAN_POINT('Ctrl Pts',(208.242953317585,-11.4401119508359,1.44118576661595));
#35391=CARTESIAN_POINT('Ctrl Pts',(208.361426469244,-10.7462948809079,-4.17975169048676));
#35392=CARTESIAN_POINT('Ctrl Pts',(208.479899620902,-7.45982377135673,-8.79228111253593));
#35393=CARTESIAN_POINT('Ctrl Pts',(208.59837277256,-2.37359354017129,-11.2835823906954));
#35394=CARTESIAN_POINT('Ctrl Pts',(208.716845924218,3.28529051715118,-11.0526034977951));
#35395=CARTESIAN_POINT('Ctrl Pts',(208.835319075877,8.15156448652971,-8.15507046465587));
#35396=CARTESIAN_POINT('Ctrl Pts',(208.953792227535,11.0511897802984,-3.29004290266605));
#35397=CARTESIAN_POINT('Ctrl Pts',(209.072265379193,11.2846020076979,2.3687413090957));
#35398=CARTESIAN_POINT('Ctrl Pts',(209.190738530852,8.79548807096082,7.4560423453157));
#35399=CARTESIAN_POINT('Ctrl Pts',(209.30921168251,4.18437227866815,10.7444965677815));
#35400=CARTESIAN_POINT('Ctrl Pts',(209.427684834168,-1.43626631304541,11.4407306121404));
#35401=CARTESIAN_POINT('Ctrl Pts',(209.546157985827,-6.71039090158305,9.37677086258944));
#35402=CARTESIAN_POINT('Ctrl Pts',(209.664631137485,-10.3655647474466,5.05056881232662));
#35403=CARTESIAN_POINT('Ctrl Pts',(209.783104289143,-11.5199396097286,-0.494134849774289));
#35404=CARTESIAN_POINT('Ctrl Pts',(209.901577440802,-9.89501069369702,-5.91962340298576));
#35405=CARTESIAN_POINT('Ctrl Pts',(210.02005059246,-5.88280879368037,-9.9169419963289));
#35406=CARTESIAN_POINT('Ctrl Pts',(210.138523744118,-0.451318836496845,
-11.5216964536208));
#35407=CARTESIAN_POINT('Ctrl Pts',(210.256996895777,5.08905642651245,-10.3467232759617));
#35408=CARTESIAN_POINT('Ctrl Pts',(210.375470047435,9.40164454536766,-6.67549681328017));
#35409=CARTESIAN_POINT('Ctrl Pts',(210.493943199093,11.4459893320066,-1.39373816520411));
#35410=CARTESIAN_POINT('Ctrl Pts',(210.612416350752,10.7288716045437,4.2242741334779));
#35411=CARTESIAN_POINT('Ctrl Pts',(210.73088950241,7.42330338187457,8.82313690034356));
#35412=CARTESIAN_POINT('Ctrl Pts',(210.849362654068,2.32678695671764,11.2933272475212));
#35413=CARTESIAN_POINT('Ctrl Pts',(210.967835805727,-3.33109072546143,11.0388863768181));
#35414=CARTESIAN_POINT('Ctrl Pts',(211.086308957385,-8.18530854892373,8.1212007622316));
#35415=CARTESIAN_POINT('Ctrl Pts',(211.204782109043,-11.0647365950617,3.24419203245698));
#35416=CARTESIAN_POINT('Ctrl Pts',(211.323255260701,-11.2746832665987,-2.41551135361317));
#35417=CARTESIAN_POINT('Ctrl Pts',(211.44172841236,-8.7644967721873,-7.4924478104204));
#35418=CARTESIAN_POINT('Ctrl Pts',(211.560201564018,-4.13978539143139,-10.7617542610137));
#35419=CARTESIAN_POINT('Ctrl Pts',(211.678674715676,1.48369174414633,-11.4346769377148));
#35420=CARTESIAN_POINT('Ctrl Pts',(211.797147867335,6.74921300408072,-9.34886633165234));
#35421=CARTESIAN_POINT('Ctrl Pts',(211.915621018993,10.3864172902835,-5.00754567963735));
#35422=CARTESIAN_POINT('Ctrl Pts',(212.034094170651,11.5177917027214,0.541896811466134));
#35423=CARTESIAN_POINT('Ctrl Pts',(212.15256732231,9.87038054147729,5.96060112975038));
#35424=CARTESIAN_POINT('Ctrl Pts',(212.271040473968,5.84163867350336,9.94124919060903));
#35425=CARTESIAN_POINT('Ctrl Pts',(212.389513625626,0.403541462807075,11.523468755082));
#35426=CARTESIAN_POINT('Ctrl Pts',(212.507986777285,-5.13191427148244,10.325533098669));
#35427=CARTESIAN_POINT('Ctrl Pts',(212.626459928943,-9.42924296622852,6.636456505198));
#35428=CARTESIAN_POINT('Ctrl Pts',(212.744933080601,-11.4516699261996,1.34626660172895));
#35429=CARTESIAN_POINT('Ctrl Pts',(212.863406232259,-10.7112638703615,-4.26872394996941));
#35430=CARTESIAN_POINT('Ctrl Pts',(212.981879383918,-7.3866553660777,-8.85384099497784));
#35431=CARTESIAN_POINT('Ctrl Pts',(213.100352535576,-2.27994036961207,-11.3028779420362));
#35432=CARTESIAN_POINT('Ctrl Pts',(213.218825687235,3.37683366346876,-11.0249794680452));
#35433=CARTESIAN_POINT('Ctrl Pts',(213.337298838893,8.21891188410895,-8.08719143478177));
#35434=CARTESIAN_POINT('Ctrl Pts',(213.455771990551,11.0780931775952,-3.1982853859645));
#35435=CARTESIAN_POINT('Ctrl Pts',(213.574245142209,11.2645706837284,2.46223986907059));
#35436=CARTESIAN_POINT('Ctrl Pts',(213.692718293868,8.73335478842003,7.52872446043392));
#35437=CARTESIAN_POINT('Ctrl Pts',(213.811191445526,4.09512733028103,10.7788269310876));
#35438=CARTESIAN_POINT('Ctrl Pts',(213.929664597184,-1.53109166664286,11.4284266708017));
#35439=CARTESIAN_POINT('Ctrl Pts',(214.048137748843,-6.78791906966887,9.32080106885565));
#35440=CARTESIAN_POINT('Ctrl Pts',(214.166610900501,-10.4070912630023,4.96443645392882));
#35441=CARTESIAN_POINT('Ctrl Pts',(214.285084052159,-11.515445774263,-0.589649456511533));
#35442=CARTESIAN_POINT('Ctrl Pts',(214.403557203818,-9.84558069118264,-6.00147637793954));
#35443=CARTESIAN_POINT('Ctrl Pts',(214.522030355476,-5.80036812003173,-9.96538546839381));
#35444=CARTESIAN_POINT('Ctrl Pts',(214.640503507134,-0.355757151167077,
-11.5250429374883));
#35445=CARTESIAN_POINT('Ctrl Pts',(214.758976658793,5.17468388520643,-10.3041653980194));
#35446=CARTESIAN_POINT('Ctrl Pts',(214.877449810451,9.4566792733418,-6.59730209879029));
#35447=CARTESIAN_POINT('Ctrl Pts',(214.995922962109,11.4571536357504,-1.29877189235286));
#35448=CARTESIAN_POINT('Ctrl Pts',(215.114396113768,10.6934719810851,4.31310037575084));
#35449=CARTESIAN_POINT('Ctrl Pts',(215.232869265426,7.34988035404288,8.88439286855379));
#35450=CARTESIAN_POINT('Ctrl Pts',(215.351342417084,2.23305458427189,11.3122343100387));
#35451=CARTESIAN_POINT('Ctrl Pts',(215.469815568742,-3.42251854473055,11.0108830105732));
#35452=CARTESIAN_POINT('Ctrl Pts',(215.588288720401,-8.25237391435474,8.05304306701711));
#35453=CARTESIAN_POINT('Ctrl Pts',(215.706761872059,-11.0912592982637,3.15232375244584));
#35454=CARTESIAN_POINT('Ctrl Pts',(215.825235023717,-11.2542644329493,-2.50892605208056));
#35455=CARTESIAN_POINT('Ctrl Pts',(215.943708175376,-8.70206265507251,-7.56487167166418));
#35456=CARTESIAN_POINT('Ctrl Pts',(216.062181327034,-4.05039886300789,-10.7957142844788));
#35457=CARTESIAN_POINT('Ctrl Pts',(216.180654478693,1.57846526560428,-11.4219799188598));
#35458=CARTESIAN_POINT('Ctrl Pts',(216.299127630351,6.8265084328873,-9.29257555671587));
#35459=CARTESIAN_POINT('Ctrl Pts',(216.417600782009,10.4275863101622,-4.92124187636331));
#35460=CARTESIAN_POINT('Ctrl Pts',(216.536073933668,11.512901864686,0.637391963915507));
#35461=CARTESIAN_POINT('Ctrl Pts',(216.654547085325,9.82061156918846,6.04224844479904));
#35462=CARTESIAN_POINT('Ctrl Pts',(216.773020236984,5.75899784281591,9.98935041471651));
#35463=CARTESIAN_POINT('Ctrl Pts',(216.891493388642,0.307966723115988,11.5264189737753));
#35464=CARTESIAN_POINT('Ctrl Pts',(217.009966540301,-5.21736453236138,10.2826205413801));
#35465=CARTESIAN_POINT('Ctrl Pts',(217.128439691959,-9.48395299500455,6.55803426722514));
#35466=CARTESIAN_POINT('Ctrl Pts',(217.246912843617,-11.4624403663795,1.25125485363602));
#35467=CARTESIAN_POINT('Ctrl Pts',(217.365385995275,-10.6754962426044,-4.35740264787347));
#35468=CARTESIAN_POINT('Ctrl Pts',(217.483859146934,-7.31297897803034,-8.91479199580349));
#35469=CARTESIAN_POINT('Ctrl Pts',(217.602332298592,-2.18613040678854,-11.3213961906678));
#35470=CARTESIAN_POINT('Ctrl Pts',(217.720805450251,3.46814458380223,-10.9965972467579));
#35471=CARTESIAN_POINT('Ctrl Pts',(217.839278601909,8.28569406435969,-8.01875624603833));
#35472=CARTESIAN_POINT('Ctrl Pts',(217.957751753567,11.104234730707,-3.1063079221047));
#35473=CARTESIAN_POINT('Ctrl Pts',(218.076224905225,11.2437646914523,2.55556909998565));
#35474=CARTESIAN_POINT('Ctrl Pts',(218.194698056884,8.6706209101412,7.60088882263999));
#35475=CARTESIAN_POINT('Ctrl Pts',(218.313171208542,4.00560075861009,10.8124160308581));
#35476=CARTESIAN_POINT('Ctrl Pts',(218.4316443602,-1.62581172654604,11.4153367927059));
#35477=CARTESIAN_POINT('Ctrl Pts',(218.550117511859,-6.86498043029599,9.26419028054612));
#35478=CARTESIAN_POINT('Ctrl Pts',(218.668590663517,-10.4479020793708,4.87796268948343));
#35479=CARTESIAN_POINT('Ctrl Pts',(218.787063815175,-11.5101600177867,-0.685123512676105));
#35480=CARTESIAN_POINT('Ctrl Pts',(218.905536966834,-9.79547360465598,-6.08291662972795));
#35481=CARTESIAN_POINT('Ctrl Pts',(219.024010118492,-5.71752855338079,-10.0131436167636));
#35482=CARTESIAN_POINT('Ctrl Pts',(219.14248327015,-0.260170999755849,-11.5275968419408));
#35483=CARTESIAN_POINT('Ctrl Pts',(219.260956421809,5.25995547801919,-10.260898895706));
#35484=CARTESIAN_POINT('Ctrl Pts',(219.379429573467,9.51106366467834,-6.51865369284798));
#35485=CARTESIAN_POINT('Ctrl Pts',(219.497902725125,11.4675300222433,-1.2037162874228));
#35486=CARTESIAN_POINT('Ctrl Pts',(219.616375876784,10.657336974314,4.40162997311355));
#35487=CARTESIAN_POINT('Ctrl Pts',(219.734849028442,7.27595185085969,8.94503792000617));
#35488=CARTESIAN_POINT('Ctrl Pts',(219.8533221801,2.13916868907181,11.3303632886701));
#35489=CARTESIAN_POINT('Ctrl Pts',(219.971795331758,-3.51371109060621,10.9821227099977));
#35490=CARTESIAN_POINT('Ctrl Pts',(220.090268483417,-8.31887156411482,7.98433096001791));
#35491=CARTESIAN_POINT('Ctrl Pts',(220.208741635075,-11.1170196637652,3.06023994245929));
#35492=CARTESIAN_POINT('Ctrl Pts',(220.327214786733,-11.2330707790818,-2.60217083598129));
#35493=CARTESIAN_POINT('Ctrl Pts',(220.445687938392,-8.639031892527,-7.6367698092379));
#35494=CARTESIAN_POINT('Ctrl Pts',(220.56416109005,-3.96073003010559,-10.828943343905));
#35495=CARTESIAN_POINT('Ctrl Pts',(220.682634241709,1.67312238226268,-11.4084734661502));
#35496=CARTESIAN_POINT('Ctrl Pts',(220.801107393367,6.9033507794017,-9.23569581394894));
#35497=CARTESIAN_POINT('Ctrl Pts',(220.919580545025,10.4680037040556,-4.83449558382035));
#35498=CARTESIAN_POINT('Ctrl Pts',(221.038053696683,11.5072892832615,0.732618747333446));
#35499=CARTESIAN_POINT('Ctrl Pts',(221.156526848342,9.7699936824466,6.12389733841086));
#35500=CARTESIAN_POINT('Ctrl Pts',(221.235508949447,7.04065173359568,8.73128281072966));
#35501=CARTESIAN_POINT('Ctrl Pts',(221.275,5.44726799658334,9.63236838871412));
#35502=CARTESIAN_POINT('Ctrl Pts',(203.669351500835,-4.88329262285739,10.2483251533871));
#35503=CARTESIAN_POINT('Ctrl Pts',(203.708842551388,-6.57856775894483,9.44053222704407));
#35504=CARTESIAN_POINT('Ctrl Pts',(203.787824652493,-9.55878961869132,6.96809332061598));
#35505=CARTESIAN_POINT('Ctrl Pts',(203.906297804152,-11.7235665905264,1.57552771572495));
#35506=CARTESIAN_POINT('Ctrl Pts',(204.02477095581,-11.0595098248454,-4.19623631507308));
#35507=CARTESIAN_POINT('Ctrl Pts',(204.143244107468,-7.72741503884474,-8.95607305850505));
#35508=CARTESIAN_POINT('Ctrl Pts',(204.261717259127,-2.53091364238729,-11.5549491457836));
#35509=CARTESIAN_POINT('Ctrl Pts',(204.380190410785,3.27615449167754,-11.3661786816061));
#35510=CARTESIAN_POINT('Ctrl Pts',(204.498663562443,8.29283689528426,-8.43515126902723));
#35511=CARTESIAN_POINT('Ctrl Pts',(204.617136714102,11.3087775377752,-3.4690806848112));
#35512=CARTESIAN_POINT('Ctrl Pts',(204.73560986576,11.5963640472022,2.33395260974631));
#35513=CARTESIAN_POINT('Ctrl Pts',(204.854083017418,9.08620638360809,7.57389042468078));
#35514=CARTESIAN_POINT('Ctrl Pts',(204.972556169076,4.38390914454991,10.986551967325));
#35515=CARTESIAN_POINT('Ctrl Pts',(205.091029320735,-1.37605171986887,11.7485937350338));
#35516=CARTESIAN_POINT('Ctrl Pts',(205.209502472393,-6.80402572759336,9.676167163528));
#35517=CARTESIAN_POINT('Ctrl Pts',(205.327975624052,-10.5904587451008,5.26926557275166));
#35518=CARTESIAN_POINT('Ctrl Pts',(205.44644877571,-11.8218347360971,-0.408900333559652));
#35519=CARTESIAN_POINT('Ctrl Pts',(205.564921927368,-10.2010716747024,-5.98841489897856));
#35520=CARTESIAN_POINT('Ctrl Pts',(205.683395079026,-6.11919526067218,-10.1231628181434));
#35521=CARTESIAN_POINT('Ctrl Pts',(205.801868230685,-0.561000131946154,
-11.8155937243948));
#35522=CARTESIAN_POINT('Ctrl Pts',(205.920341382343,5.13254204483568,-10.6573912526731));
#35523=CARTESIAN_POINT('Ctrl Pts',(206.038814534001,9.58780572390719,-6.92798365839843));
#35524=CARTESIAN_POINT('Ctrl Pts',(206.15728768566,11.7299127746237,-1.52712883183816));
#35525=CARTESIAN_POINT('Ctrl Pts',(206.275760837318,11.0420578635646,4.24216151322699));
#35526=CARTESIAN_POINT('Ctrl Pts',(206.394233988976,7.69019305501607,8.98798681272517));
#35527=CARTESIAN_POINT('Ctrl Pts',(206.512707140635,2.48299016843104,11.5653679574455));
#35528=CARTESIAN_POINT('Ctrl Pts',(206.631180292293,-3.32325960468488,11.3524852683539));
#35529=CARTESIAN_POINT('Ctrl Pts',(206.749653443951,-8.32773885743942,8.40069888106815));
#35530=CARTESIAN_POINT('Ctrl Pts',(206.86812659561,-11.323065557707,3.42215758608464));
#35531=CARTESIAN_POINT('Ctrl Pts',(206.986599747268,-11.5865863672557,-2.38201438330499));
#35532=CARTESIAN_POINT('Ctrl Pts',(207.105072898926,-9.05472418355536,-7.61150091163746));
#35533=CARTESIAN_POINT('Ctrl Pts',(207.223546050585,-4.33831676893397,-11.0046346500247));
#35534=CARTESIAN_POINT('Ctrl Pts',(207.342019202243,1.4247541348989,-11.7427872254937));
#35535=CARTESIAN_POINT('Ctrl Pts',(207.460492353901,6.84408846680124,-9.6478717459723));
#35536=CARTESIAN_POINT('Ctrl Pts',(207.578965505559,10.6122161449094,-5.2253080925297));
#35537=CARTESIAN_POINT('Ctrl Pts',(207.697438657218,11.8200376558811,0.457914819243914));
#35538=CARTESIAN_POINT('Ctrl Pts',(207.815911808876,10.1761536519165,6.03066107659177));
#35539=CARTESIAN_POINT('Ctrl Pts',(207.934384960534,6.07716803703832,10.1484483945937));
#35540=CARTESIAN_POINT('Ctrl Pts',(208.052858112193,0.512003200827929,11.8178182796349));
#35541=CARTESIAN_POINT('Ctrl Pts',(208.171331263851,-5.17668766753006,10.6360180970593));
#35542=CARTESIAN_POINT('Ctrl Pts',(208.289804415509,-9.6164494545789,6.88816928186734));
#35543=CARTESIAN_POINT('Ctrl Pts',(208.408277567168,-11.7361440183151,1.47847886339215));
#35544=CARTESIAN_POINT('Ctrl Pts',(208.526750718826,-11.0243732690398,-4.28790976969105));
#35545=CARTESIAN_POINT('Ctrl Pts',(208.645223870484,-7.65285921222969,-9.01979611997538));
#35546=CARTESIAN_POINT('Ctrl Pts',(208.763697022143,-2.43501425056925,-11.5755639935018));
#35547=CARTESIAN_POINT('Ctrl Pts',(208.882170173801,3.37030291460337,-11.3386081346851));
#35548=CARTESIAN_POINT('Ctrl Pts',(209.000643325459,8.36249987759127,-8.3660965787766));
#35549=CARTESIAN_POINT('Ctrl Pts',(209.119116477118,11.3371578348792,-3.37517827605727));
#35550=CARTESIAN_POINT('Ctrl Pts',(209.237589628776,11.5766099948028,2.43003645988342));
#35551=CARTESIAN_POINT('Ctrl Pts',(209.356062780434,9.02308606382359,7.6489799354531));
#35552=CARTESIAN_POINT('Ctrl Pts',(209.474535932093,4.2926499233346,11.0225284215477));
#35553=CARTESIAN_POINT('Ctrl Pts',(209.593009083751,-1.47343211071668,11.7367786885176));
#35554=CARTESIAN_POINT('Ctrl Pts',(209.711482235409,-6.88403351108953,9.6194105217694));
#35555=CARTESIAN_POINT('Ctrl Pts',(209.829955387068,-10.6337911053672,5.1812607438291));
#35556=CARTESIAN_POINT('Ctrl Pts',(209.948428538726,-11.8180373516528,-0.506921417057956));
#35557=CARTESIAN_POINT('Ctrl Pts',(210.066901690384,-10.1510606769466,-6.07280357833852));
#35558=CARTESIAN_POINT('Ctrl Pts',(210.185374842043,-6.03503632932535,-10.1735594887854));
#35559=CARTESIAN_POINT('Ctrl Pts',(210.303847993701,-0.462997467688116,
-11.8198396568247));
#35560=CARTESIAN_POINT('Ctrl Pts',(210.422321145359,5.22074428952753,-10.614462079234));
#35561=CARTESIAN_POINT('Ctrl Pts',(210.540794297017,9.64492785277154,-6.84823647977811));
#35562=CARTESIAN_POINT('Ctrl Pts',(210.659267448676,11.7421734865726,-1.42980347578353));
#35563=CARTESIAN_POINT('Ctrl Pts',(210.777740600334,11.0064991362026,4.33358430550301));
#35564=CARTESIAN_POINT('Ctrl Pts',(210.896213751992,7.61539379647069,9.05145035299908));
#35565=CARTESIAN_POINT('Ctrl Pts',(211.014686903651,2.38699646833266,11.5855610148278));
#35566=CARTESIAN_POINT('Ctrl Pts',(211.133160055309,-3.41728828005328,11.3245360602164));
#35567=CARTESIAN_POINT('Ctrl Pts',(211.251633206967,-8.3971171241463,8.33135044104499));
#35568=CARTESIAN_POINT('Ctrl Pts',(211.370106358626,-11.3510551961755,3.32814093774701));
#35569=CARTESIAN_POINT('Ctrl Pts',(211.488579510284,-11.5664345896564,-2.47801675767762));
#35570=CARTESIAN_POINT('Ctrl Pts',(211.607052661942,-8.99129281326067,-7.68632745297379));
#35571=CARTESIAN_POINT('Ctrl Pts',(211.725525813601,-4.24690927567419,-11.0402326865118));
#35572=CARTESIAN_POINT('Ctrl Pts',(211.843998965259,1.52208475432044,-11.7305683651218));
#35573=CARTESIAN_POINT('Ctrl Pts',(211.962472116917,6.9238602005454,-9.59078391433333));
#35574=CARTESIAN_POINT('Ctrl Pts',(212.080945268576,10.6551832426936,-5.13712431548555));
#35575=CARTESIAN_POINT('Ctrl Pts',(212.199418420234,11.8158338639524,0.555919299545619));
#35576=CARTESIAN_POINT('Ctrl Pts',(212.317891571892,10.1257931782642,6.11484167245154));
#35577=CARTESIAN_POINT('Ctrl Pts',(212.43636472355,5.99280086329799,10.1984956724502));
#35578=CARTESIAN_POINT('Ctrl Pts',(212.554837875209,0.413983774391252,11.8216578195561));
#35579=CARTESIAN_POINT('Ctrl Pts',(212.673311026867,-5.26471115305508,10.5927235705945));
#35580=CARTESIAN_POINT('Ctrl Pts',(212.791784178525,-9.67324042902019,6.80818593830257));
#35581=CARTESIAN_POINT('Ctrl Pts',(212.910257330184,-11.7480010756596,1.38110350605304));
#35582=CARTESIAN_POINT('Ctrl Pts',(213.028730481842,-10.9884357723924,-4.37918433548295));
#35583=CARTESIAN_POINT('Ctrl Pts',(213.1472036335,-7.5777974518522,-9.08294896753436));
#35584=CARTESIAN_POINT('Ctrl Pts',(213.265676785159,-2.33893764728264,-11.595358849568));
#35585=CARTESIAN_POINT('Ctrl Pts',(213.384149936817,3.46421489323522,-11.3102692868746));
#35586=CARTESIAN_POINT('Ctrl Pts',(213.502623088475,8.43159000194017,-8.29646106525633));
#35587=CARTESIAN_POINT('Ctrl Pts',(213.621096240134,11.3647574026644,-3.28104637984854));
#35588=CARTESIAN_POINT('Ctrl Pts',(213.739569391792,11.5560603267582,2.52595445177774));
#35589=CARTESIAN_POINT('Ctrl Pts',(213.85804254345,8.9593449784773,7.72354282209696));
#35590=CARTESIAN_POINT('Ctrl Pts',(213.976515695109,4.20109561235587,11.0577471405335));
#35591=CARTESIAN_POINT('Ctrl Pts',(214.094988846767,-1.57071122924191,11.7241563620785));
#35592=CARTESIAN_POINT('Ctrl Pts',(214.213461998425,-6.96356785044228,9.56199241583145));
#35593=CARTESIAN_POINT('Ctrl Pts',(214.331935150084,-10.6763921891008,5.09289956632158));
#35594=CARTESIAN_POINT('Ctrl Pts',(214.450408301742,-11.8134272306639,-0.604907624302995));
#35595=CARTESIAN_POINT('Ctrl Pts',(214.5688814534,-10.1003515902849,-6.15677463618423));
#35596=CARTESIAN_POINT('Ctrl Pts',(214.687354605058,-5.95046236509621,-10.223256516869));
#35597=CARTESIAN_POINT('Ctrl Pts',(214.805827756717,-0.364962963613078,
-11.8232727365701));
#35598=CARTESIAN_POINT('Ctrl Pts',(214.924300908375,5.3085875022053,-10.5708029448837));
#35599=CARTESIAN_POINT('Ctrl Pts',(215.042774060034,9.70138669655638,-6.76801834601613));
#35600=CARTESIAN_POINT('Ctrl Pts',(215.161247211692,11.7536266853844,-1.33237979148266));
#35601=CARTESIAN_POINT('Ctrl Pts',(215.27972036335,10.9701834881662,4.42470907564521));
#35602=CARTESIAN_POINT('Ctrl Pts',(215.398193515008,7.54007082475531,9.11429142203635));
#35603=CARTESIAN_POINT('Ctrl Pts',(215.516666666667,2.290838613678,11.6049573292716));
#35604=CARTESIAN_POINT('Ctrl Pts',(215.635139818325,-3.51108194735603,11.2958080599434));
#35605=CARTESIAN_POINT('Ctrl Pts',(215.753612969983,-8.46591791829252,8.26142905125167));
#35606=CARTESIAN_POINT('Ctrl Pts',(215.872086121641,-11.3782642187683,3.23389541204245));
#35607=CARTESIAN_POINT('Ctrl Pts',(215.9905592733,-11.5454873844695,-2.5738487180074));
#35608=CARTESIAN_POINT('Ctrl Pts',(216.109032424958,-8.92724310874166,-7.76062540299144));
#35609=CARTESIAN_POINT('Ctrl Pts',(216.227505576617,-4.15520972103837,-11.0750714824926));
#35610=CARTESIAN_POINT('Ctrl Pts',(216.345978728275,1.6193106994627,-11.7175427896269));
#35611=CARTESIAN_POINT('Ctrl Pts',(216.464451879933,7.00315577810006,-9.5330365212662));
#35612=CARTESIAN_POINT('Ctrl Pts',(216.582925031591,10.6974175799506,-5.04858725667831));
#35613=CARTESIAN_POINT('Ctrl Pts',(216.70139818325,11.8108174931637,0.653885549090481));
#35614=CARTESIAN_POINT('Ctrl Pts',(216.819871334908,10.0747363504171,6.19860174859746));
#35615=CARTESIAN_POINT('Ctrl Pts',(216.938344486567,5.90802156263124,10.2478415963371));
#35616=CARTESIAN_POINT('Ctrl Pts',(217.056817638225,0.315935878151426,11.824684380102));
#35617=CARTESIAN_POINT('Ctrl Pts',(217.175290789883,-5.35237258262742,10.5487005789751));
#35618=CARTESIAN_POINT('Ctrl Pts',(217.293763941541,-9.72936617147105,6.72773439350622));
#35619=CARTESIAN_POINT('Ctrl Pts',(217.4122370932,-11.7590502190278,1.28363316976241));
#35620=CARTESIAN_POINT('Ctrl Pts',(217.530710244858,-10.9517425973294,-4.47015774329848));
#35621=CARTESIAN_POINT('Ctrl Pts',(217.649183396516,-7.50221456380103,-9.14547717764492));
#35622=CARTESIAN_POINT('Ctrl Pts',(217.767656548175,-2.24270019446914,-11.6143562889149));
#35623=CARTESIAN_POINT('Ctrl Pts',(217.886129699833,3.55788863664646,-11.28115262805));
#35624=CARTESIAN_POINT('Ctrl Pts',(218.004602851491,8.50010028301504,-8.22625500132398));
#35625=CARTESIAN_POINT('Ctrl Pts',(218.12307600315,11.3915754122696,-3.18668884498026));
#35626=CARTESIAN_POINT('Ctrl Pts',(218.241549154808,11.5347159445663,2.62169873293905));
#35627=CARTESIAN_POINT('Ctrl Pts',(218.360022306466,8.8949877559718,7.79757455810444));
#35628=CARTESIAN_POINT('Ctrl Pts',(218.478495458124,4.10925239061891,11.0922054145474));
#35629=CARTESIAN_POINT('Ctrl Pts',(218.596968609783,-1.66788232942209,11.7107277614516));
#35630=CARTESIAN_POINT('Ctrl Pts',(218.715441761441,-7.0426233029111,9.50391672850897));
#35631=CARTESIAN_POINT('Ctrl Pts',(218.8339149131,-10.7182590537316,5.00418814831287));
#35632=CARTESIAN_POINT('Ctrl Pts',(218.952388064758,-11.8080046963812,-0.702852231661334));
#35633=CARTESIAN_POINT('Ctrl Pts',(219.070861216416,-10.0489478989274,-6.24032229096106));
#35634=CARTESIAN_POINT('Ctrl Pts',(219.189334368075,-5.86547918583989,-10.2722504873586));
#35635=CARTESIAN_POINT('Ctrl Pts',(219.307807519733,-0.266903360355729,
-11.8258927275801));
#35636=CARTESIAN_POINT('Ctrl Pts',(219.426280671391,5.39606564037585,-10.5264168493191));
#35637=CARTESIAN_POINT('Ctrl Pts',(219.544753823049,9.75717837515331,-6.68733478077511));
#35638=CARTESIAN_POINT('Ctrl Pts',(219.663226974708,11.764271578266,-1.23486446348573));
#35639=CARTESIAN_POINT('Ctrl Pts',(219.781700126366,10.9331134275417,4.51552952469302));
#35640=CARTESIAN_POINT('Ctrl Pts',(219.900173278024,7.46422929766668,9.17650576582092));
#35641=CARTESIAN_POINT('Ctrl Pts',(220.018646429683,2.19452326361045,11.6235554256046));
#35642=CARTESIAN_POINT('Ctrl Pts',(220.137119581341,-3.604634253172,11.2663035383954));
#35643=CARTESIAN_POINT('Ctrl Pts',(220.255592732999,-8.5341363061735,8.19093890333965));
#35644=CARTESIAN_POINT('Ctrl Pts',(220.374065884658,-11.404691176895,3.13942877916317));
#35645=CARTESIAN_POINT('Ctrl Pts',(220.492539036316,-11.5237453092929,-2.66950636694637));
#35646=CARTESIAN_POINT('Ctrl Pts',(220.611012187974,-8.86258131959157,-7.83438402535808));
#35647=CARTESIAN_POINT('Ctrl Pts',(220.729485339632,-4.06322055682231,-11.109160399515));
#35648=CARTESIAN_POINT('Ctrl Pts',(220.847958491291,1.71641722763616,-11.7036868348201));
#35649=CARTESIAN_POINT('Ctrl Pts',(220.966431642949,7.08198654909897,-9.47468491983902));
#35650=CARTESIAN_POINT('Ctrl Pts',(221.084904794608,10.7388808416404,-4.95959625845083));
#35651=CARTESIAN_POINT('Ctrl Pts',(221.203377946266,11.8050596767895,0.751576485105512));
#35652=CARTESIAN_POINT('Ctrl Pts',(221.321851097924,10.022808641033,6.2823634441545));
#35653=CARTESIAN_POINT('Ctrl Pts',(221.40083319903,7.22284039556463,8.95721938489205));
#35654=CARTESIAN_POINT('Ctrl Pts',(221.440324249582,5.58822518424655,9.88162206219974));
#35655=CARTESIAN_POINT('Ctrl Pts',(203.834675750418,-5.00646861737437,10.506828532233));
#35656=CARTESIAN_POINT('Ctrl Pts',(203.87416680097,-6.74450531149134,9.6786598666602));
#35657=CARTESIAN_POINT('Ctrl Pts',(203.953148902076,-9.79990017842918,7.14385625168357));
#35658=CARTESIAN_POINT('Ctrl Pts',(204.071622053734,-12.0192814054271,1.61526876920292));
#35659=CARTESIAN_POINT('Ctrl Pts',(204.190095205392,-11.3384744961758,-4.30208202641095));
#35660=CARTESIAN_POINT('Ctrl Pts',(204.308568357051,-7.92233107316142,-9.18198071777258));
#35661=CARTESIAN_POINT('Ctrl Pts',(204.427041508709,-2.59475331553703,-11.8464107604251));
#35662=CARTESIAN_POINT('Ctrl Pts',(204.545514660367,3.35879209275325,-11.6528787569633));
#35663=CARTESIAN_POINT('Ctrl Pts',(204.663987812026,8.50201510982795,-8.64791921612924));
#35664=CARTESIAN_POINT('Ctrl Pts',(204.782460963684,11.5940297287798,-3.55658464912643));
#35665=CARTESIAN_POINT('Ctrl Pts',(204.900934115342,11.8888703098024,2.39282414501235));
#35666=CARTESIAN_POINT('Ctrl Pts',(205.019407267001,9.31539652110854,7.76493395974479));
#35667=CARTESIAN_POINT('Ctrl Pts',(205.137880418659,4.49448870847458,11.2636763523257));
#35668=CARTESIAN_POINT('Ctrl Pts',(205.256353570317,-1.41076119812299,12.0449398337123));
#35669=CARTESIAN_POINT('Ctrl Pts',(205.374826721975,-6.97565022369513,9.92023845016386));
#35670=CARTESIAN_POINT('Ctrl Pts',(205.493299873634,-10.8575920891509,5.40217733484019));
#35671=CARTESIAN_POINT('Ctrl Pts',(205.611773025292,-12.1200282631076,-0.419214420618188));
#35672=CARTESIAN_POINT('Ctrl Pts',(205.730246176951,-10.4583831335302,-6.13946645736958));
#35673=CARTESIAN_POINT('Ctrl Pts',(205.848719328609,-6.27354561812342,-10.3785091068229));
#35674=CARTESIAN_POINT('Ctrl Pts',(205.967192480267,-0.575150778756315,
-12.1136298283544));
#35675=CARTESIAN_POINT('Ctrl Pts',(206.085665631925,5.26200509765657,-10.9262128998462));
#35676=CARTESIAN_POINT('Ctrl Pts',(206.204138783584,9.82964818482179,-7.10273486481322));
#35677=CARTESIAN_POINT('Ctrl Pts',(206.322611935242,12.02578766544,-1.56564907363911));
#35678=CARTESIAN_POINT('Ctrl Pts',(206.441085086901,11.320582327262,4.34916564008343));
#35679=CARTESIAN_POINT('Ctrl Pts',(206.559558238559,7.88417020337402,9.21469946336195));
#35680=CARTESIAN_POINT('Ctrl Pts',(206.678031390217,2.54562102162646,11.8570923758113));
#35681=CARTESIAN_POINT('Ctrl Pts',(206.796504541875,-3.40708538340826,11.6388399415561));
#35682=CARTESIAN_POINT('Ctrl Pts',(206.914977693534,-8.53779743780001,8.61259780239634));
#35683=CARTESIAN_POINT('Ctrl Pts',(207.033450845192,-11.6086781492038,3.50847796387377));
#35684=CARTESIAN_POINT('Ctrl Pts',(207.15192399685,-11.8788459980145,-2.44209822698946));
#35685=CARTESIAN_POINT('Ctrl Pts',(207.270397148509,-9.28312021519312,-7.8034931322489));
#35686=CARTESIAN_POINT('Ctrl Pts',(207.388870300167,-4.4477463124436,-11.2822151519525));
#35687=CARTESIAN_POINT('Ctrl Pts',(207.507343451825,1.46069208108849,-12.0389868609878));
#35688=CARTESIAN_POINT('Ctrl Pts',(207.625816603484,7.01672350397154,-9.89122931003062));
#35689=CARTESIAN_POINT('Ctrl Pts',(207.744289755142,10.8798982968165,-5.35711107274481));
#35690=CARTESIAN_POINT('Ctrl Pts',(207.8627629068,12.118185853406,0.469465245896696));
#35691=CARTESIAN_POINT('Ctrl Pts',(207.981236058459,10.4328365794489,6.18277825102179));
#35692=CARTESIAN_POINT('Ctrl Pts',(208.099709210117,6.23045830133773,10.4044324857287));
#35693=CARTESIAN_POINT('Ctrl Pts',(208.218182361775,0.524917950839583,12.1159104956945));
#35694=CARTESIAN_POINT('Ctrl Pts',(208.336655513434,-5.30726424792321,10.9043006285369));
#35695=CARTESIAN_POINT('Ctrl Pts',(208.455128665092,-9.85901442390833,7.06191621190467));
#35696=CARTESIAN_POINT('Ctrl Pts',(208.57360181675,-12.0321760857944,1.51577196016836));
#35697=CARTESIAN_POINT('Ctrl Pts',(208.692074968408,-11.3024516571717,-4.39606784889534));
#35698=CARTESIAN_POINT('Ctrl Pts',(208.810548120067,-7.84589465310265,-9.24731112741483));
#35699=CARTESIAN_POINT('Ctrl Pts',(208.929021271725,-2.49643496096719,-11.8675455963083));
#35700=CARTESIAN_POINT('Ctrl Pts',(209.047494423383,3.45531531205556,-11.6246127715752));
#35701=CARTESIAN_POINT('Ctrl Pts',(209.165967575042,8.57343526865283,-8.57712269289734));
#35702=CARTESIAN_POINT('Ctrl Pts',(209.2844407267,11.62312588946,-3.46031364944849));
#35703=CARTESIAN_POINT('Ctrl Pts',(209.402913878358,11.8686179819078,2.49133161067114));
#35704=CARTESIAN_POINT('Ctrl Pts',(209.521387030017,9.25068405668635,7.84191752559052));
#35705=CARTESIAN_POINT('Ctrl Pts',(209.639860181675,4.40092756800106,11.3005602753139));
#35706=CARTESIAN_POINT('Ctrl Pts',(209.758333333333,-1.51059790838795,12.0328267648948));
#35707=CARTESIAN_POINT('Ctrl Pts',(209.876806484992,-7.05767612059601,9.86205018094938));
#35708=CARTESIAN_POINT('Ctrl Pts',(209.99527963665,-10.9020174632878,5.31195267533158));
#35709=CARTESIAN_POINT('Ctrl Pts',(210.113752788308,-12.1161350935769,-0.519707984341627));
#35710=CARTESIAN_POINT('Ctrl Pts',(210.232225939967,-10.4071106601961,-6.22598375369127));
#35711=CARTESIAN_POINT('Ctrl Pts',(210.350699091625,-6.18726386497032,-10.4301769812418));
#35712=CARTESIAN_POINT('Ctrl Pts',(210.469172243283,-0.474676098879385,
-12.1179828600286));
#35713=CARTESIAN_POINT('Ctrl Pts',(210.587645394941,5.3524321525426,-10.8822008825064));
#35714=CARTESIAN_POINT('Ctrl Pts',(210.7061185466,9.88821116017542,-7.02097614627605));
#35715=CARTESIAN_POINT('Ctrl Pts',(210.824591698258,12.0383576411386,-1.46586878636295));
#35716=CARTESIAN_POINT('Ctrl Pts',(210.943064849916,11.2841266678616,4.44289447752812));
#35717=CARTESIAN_POINT('Ctrl Pts',(211.061538001575,7.8074842110668,9.27976380565459));
#35718=CARTESIAN_POINT('Ctrl Pts',(211.180011153233,2.44720597994769,11.8777947821346));
#35719=CARTESIAN_POINT('Ctrl Pts',(211.298484304891,-3.50348583464514,11.6101857436148));
#35720=CARTESIAN_POINT('Ctrl Pts',(211.41695745655,-8.60892569936886,8.54150011985839));
#35721=CARTESIAN_POINT('Ctrl Pts',(211.535430608208,-11.6373737972894,3.41208984303704));
#35722=CARTESIAN_POINT('Ctrl Pts',(211.653903759866,-11.8581859127141,-2.54052216174207));
#35723=CARTESIAN_POINT('Ctrl Pts',(211.772376911525,-9.21808885433405,-7.88020709552718));
#35724=CARTESIAN_POINT('Ctrl Pts',(211.890850063183,-4.35403315991698,-11.31871111201));
#35725=CARTESIAN_POINT('Ctrl Pts',(212.009323214841,1.56047776449454,-12.0264597925288));
#35726=CARTESIAN_POINT('Ctrl Pts',(212.1277963665,7.09850739701008,-9.83270149701432));
#35727=CARTESIAN_POINT('Ctrl Pts',(212.246269518158,10.9239491951037,-5.26670295133374));
#35728=CARTESIAN_POINT('Ctrl Pts',(212.364742669816,12.1138760251834,0.569941787625099));
#35729=CARTESIAN_POINT('Ctrl Pts',(212.483215821475,10.3812058150511,6.2690822151527));
#35730=CARTESIAN_POINT('Ctrl Pts',(212.601688973133,6.14396305309261,10.4557421542915));
#35731=CARTESIAN_POINT('Ctrl Pts',(212.720162124791,0.424426085975434,12.1198468840303));
#35732=CARTESIAN_POINT('Ctrl Pts',(212.83863527645,-5.39750803462773,10.85991404252));
#35733=CARTESIAN_POINT('Ctrl Pts',(212.957108428108,-9.91723789181186,6.97991537140715));
#35734=CARTESIAN_POINT('Ctrl Pts',(213.075581579766,-12.0443322251196,1.41594041037714));
#35735=CARTESIAN_POINT('Ctrl Pts',(213.194054731424,-11.2656076744232,-4.48964472099649));
#35736=CARTESIAN_POINT('Ctrl Pts',(213.312527883083,-7.76893953762672,-9.31205694009088));
#35737=CARTESIAN_POINT('Ctrl Pts',(213.431001034741,-2.3979349249532,-11.8878397570999));
#35738=CARTESIAN_POINT('Ctrl Pts',(213.5494741864,3.55159612300168,-11.595559105704));
#35739=CARTESIAN_POINT('Ctrl Pts',(213.667947338058,8.6442681197714,-8.50573069573088));
#35740=CARTESIAN_POINT('Ctrl Pts',(213.786420489716,11.6514216277335,-3.36380737373258));
#35741=CARTESIAN_POINT('Ctrl Pts',(213.904893641374,11.847549969788,2.58966903448489));
#35742=CARTESIAN_POINT('Ctrl Pts',(214.023366793033,9.18533516853456,7.91836118376));
#35743=CARTESIAN_POINT('Ctrl Pts',(214.141839944691,4.30706389443071,11.3366673499793));
#35744=CARTESIAN_POINT('Ctrl Pts',(214.260313096349,-1.61033079184096,12.0198860533552));
#35745=CARTESIAN_POINT('Ctrl Pts',(214.378786248007,-7.1392166312157,9.80318376280727));
#35746=CARTESIAN_POINT('Ctrl Pts',(214.497259399666,-10.9456931151994,5.22136267871434));
#35747=CARTESIAN_POINT('Ctrl Pts',(214.615732551324,-12.1114086870649,-0.620165792094453));
#35748=CARTESIAN_POINT('Ctrl Pts',(214.734205702983,-10.3551224893871,-6.31207289442892));
#35749=CARTESIAN_POINT('Ctrl Pts',(214.852678854641,-6.10055661016068,-10.4811275653443));
#35750=CARTESIAN_POINT('Ctrl Pts',(214.971152006299,-0.374168776059084,
-12.121502535652));
#35751=CARTESIAN_POINT('Ctrl Pts',(215.089625157957,5.44249111920418,-10.837440491748));
#35752=CARTESIAN_POINT('Ctrl Pts',(215.208098309616,9.94609411977095,-6.93873459324197));
#35753=CARTESIAN_POINT('Ctrl Pts',(215.326571461274,12.0500997350184,-1.36598769061246));
#35754=CARTESIAN_POINT('Ctrl Pts',(215.445044612933,11.2468949952473,4.53631777553957));
#35755=CARTESIAN_POINT('Ctrl Pts',(215.563517764591,7.73026129546775,9.3441899755189));
#35756=CARTESIAN_POINT('Ctrl Pts',(215.681990916249,2.34862264308409,11.8976803485044));
#35757=CARTESIAN_POINT('Ctrl Pts',(215.800464067907,-3.59964534998152,11.5807331093136));
#35758=CARTESIAN_POINT('Ctrl Pts',(215.918937219566,-8.67946192223031,8.46981503548623));
#35759=CARTESIAN_POINT('Ctrl Pts',(216.037410371224,-11.6652691392729,3.31546707163905));
#35760=CARTESIAN_POINT('Ctrl Pts',(216.155883522882,-11.8367103359897,-2.63877138393424));
#35761=CARTESIAN_POINT('Ctrl Pts',(216.27435667454,-9.15242356241081,-7.95637913431871));
#35762=CARTESIAN_POINT('Ctrl Pts',(216.392829826199,-4.26002057906886,-11.3544286805063));
#35763=CARTESIAN_POINT('Ctrl Pts',(216.511302977857,1.66015613332113,-12.013105660394));
#35764=CARTESIAN_POINT('Ctrl Pts',(216.629776129516,7.17980312331282,-9.77349748581652));
#35765=CARTESIAN_POINT('Ctrl Pts',(216.748249281174,10.967248849739,-5.17593263699331));
#35766=CARTESIAN_POINT('Ctrl Pts',(216.866722432832,12.1087331216414,0.670379134265463));
#35767=CARTESIAN_POINT('Ctrl Pts',(216.98519558449,10.3288611316458,6.35495505239587));
#35768=CARTESIAN_POINT('Ctrl Pts',(217.103668736149,6.05704528244657,10.5063327779576));
#35769=CARTESIAN_POINT('Ctrl Pts',(217.222141887807,0.323905033186873,12.1229497864287));
#35770=CARTESIAN_POINT('Ctrl Pts',(217.340615039465,-5.48738063289348,10.8147806165701));
#35771=CARTESIAN_POINT('Ctrl Pts',(217.459088191124,-9.97477934793755,6.89743451978729));
#35772=CARTESIAN_POINT('Ctrl Pts',(217.577561342782,-12.055660071676,1.31601148588881));
#35773=CARTESIAN_POINT('Ctrl Pts',(217.69603449444,-11.2279889520545,-4.5829128387235));
#35774=CARTESIAN_POINT('Ctrl Pts',(217.814507646099,-7.69145014957172,-9.37616235948635));
#35775=CARTESIAN_POINT('Ctrl Pts',(217.932980797757,-2.29926998214972,-11.907316387162));
#35776=CARTESIAN_POINT('Ctrl Pts',(218.051453949415,3.64763268949068,-11.5657080093421));
#35777=CARTESIAN_POINT('Ctrl Pts',(218.169927101074,8.71450650167041,-8.43375375660963));
#35778=CARTESIAN_POINT('Ctrl Pts',(218.288400252732,11.6789160938322,-3.26706976785583));
#35779=CARTESIAN_POINT('Ctrl Pts',(218.40687340439,11.8256671976804,2.68782836589246));
#35780=CARTESIAN_POINT('Ctrl Pts',(218.525346556049,9.11935460180238,7.9942602935689));
#35781=CARTESIAN_POINT('Ctrl Pts',(218.643819707707,4.21290402262775,11.3719947982367));
#35782=CARTESIAN_POINT('Ctrl Pts',(218.762292859365,-1.70995293229815,12.0061187301973));
#35783=CARTESIAN_POINT('Ctrl Pts',(218.880766011024,-7.2202661755262,9.74364317647182));
#35784=CARTESIAN_POINT('Ctrl Pts',(218.999239162682,-10.9886160280923,5.13041360714233));
#35785=CARTESIAN_POINT('Ctrl Pts',(219.11771231434,-12.1058493749757,-0.720580950646571));
#35786=CARTESIAN_POINT('Ctrl Pts',(219.236185465999,-10.3024221931989,-6.39772795219415));
#35787=CARTESIAN_POINT('Ctrl Pts',(219.354658617657,-6.01342981829898,-10.5313573579535));
#35788=CARTESIAN_POINT('Ctrl Pts',(219.473131769315,-0.273635720955611,
-12.1241886132193));
#35789=CARTESIAN_POINT('Ctrl Pts',(219.591604920973,5.5321758027325,-10.7919348029323));
#35790=CARTESIAN_POINT('Ctrl Pts',(219.710078072632,10.0032930856283,-6.85601586870224));
#35791=CARTESIAN_POINT('Ctrl Pts',(219.82855122429,12.0610131342887,-1.26601263954867));
#35792=CARTESIAN_POINT('Ctrl Pts',(219.947024375948,11.2088898807694,4.6294290762725));
#35793=CARTESIAN_POINT('Ctrl Pts',(220.065497527607,7.65250674447366,9.40797361163566));
#35794=CARTESIAN_POINT('Ctrl Pts',(220.183970679265,2.24987783814909,11.9167475625392));
#35795=CARTESIAN_POINT('Ctrl Pts',(220.302443830923,-3.69555741573779,11.5504843667932));
#35796=CARTESIAN_POINT('Ctrl Pts',(220.420916982582,-8.74940104823217,8.39754684666139));
#35797=CARTESIAN_POINT('Ctrl Pts',(220.53939013424,-11.6923626900249,3.21861761586706));
#35798=CARTESIAN_POINT('Ctrl Pts',(220.657863285898,-11.8144198395041,-2.73684189791147));
#35799=CARTESIAN_POINT('Ctrl Pts',(220.776336437557,-9.08613074665614,-8.03199824147826));
#35800=CARTESIAN_POINT('Ctrl Pts',(220.894809589215,-4.16571108353903,-11.3893774551249));
#35801=CARTESIAN_POINT('Ctrl Pts',(221.013282740873,1.75971207300965,-11.9989002034899));
#35802=CARTESIAN_POINT('Ctrl Pts',(221.131755892532,7.26062231879625,-9.71367402572911));
#35803=CARTESIAN_POINT('Ctrl Pts',(221.25022904419,11.0097579792252,-5.0846969330813));
#35804=CARTESIAN_POINT('Ctrl Pts',(221.368702195848,12.1028300703176,0.770534222877572));
#35805=CARTESIAN_POINT('Ctrl Pts',(221.487175347506,10.2756235996193,6.44082954989814));
#35806=CARTESIAN_POINT('Ctrl Pts',(221.566157448612,7.40502905753358,9.18315595905444));
#35807=CARTESIAN_POINT('Ctrl Pts',(221.605648499165,5.72918237190977,10.1308757356854));
#35808=CARTESIAN_POINT('Ctrl Pts',(204.,-5.12964461189134,10.7653319110789));
#35809=CARTESIAN_POINT('Ctrl Pts',(204.039491050553,-6.91044286403785,9.91678750627633));
#35810=CARTESIAN_POINT('Ctrl Pts',(204.118473151658,-10.041010738167,7.31961918275114));
#35811=CARTESIAN_POINT('Ctrl Pts',(204.236946303317,-12.3149962203278,1.65500982268089));
#35812=CARTESIAN_POINT('Ctrl Pts',(204.355419454975,-11.6174391675063,-4.40792773774884));
#35813=CARTESIAN_POINT('Ctrl Pts',(204.473892606633,-8.11724710747811,-9.40788837704011));
#35814=CARTESIAN_POINT('Ctrl Pts',(204.592365758292,-2.65859298868677,-12.1378723750666));
#35815=CARTESIAN_POINT('Ctrl Pts',(204.71083890995,3.44142969382895,-11.9395788323205));
#35816=CARTESIAN_POINT('Ctrl Pts',(204.829312061608,8.71119332437167,-8.86068716323123));
#35817=CARTESIAN_POINT('Ctrl Pts',(204.947785213267,11.8792819197844,-3.64408861344167));
#35818=CARTESIAN_POINT('Ctrl Pts',(205.066258364925,12.1813765724026,2.4516956802784));
#35819=CARTESIAN_POINT('Ctrl Pts',(205.184731516583,9.54458665860898,7.9559774948088));
#35820=CARTESIAN_POINT('Ctrl Pts',(205.303204668241,4.60506827239925,11.5408007373264));
#35821=CARTESIAN_POINT('Ctrl Pts',(205.4216778199,-1.44547067637712,12.3412859323907));
#35822=CARTESIAN_POINT('Ctrl Pts',(205.540150971558,-7.14727471979692,10.1643097367997));
#35823=CARTESIAN_POINT('Ctrl Pts',(205.658624123217,-11.1247254332009,5.53508909692871));
#35824=CARTESIAN_POINT('Ctrl Pts',(205.777097274875,-12.4182217901181,-0.429528507676729));
#35825=CARTESIAN_POINT('Ctrl Pts',(205.895570426533,-10.715694592358,-6.2905180157606));
#35826=CARTESIAN_POINT('Ctrl Pts',(206.014043578191,-6.42789597557465,-10.6338553955023));
#35827=CARTESIAN_POINT('Ctrl Pts',(206.13251672985,-0.589301425566469,-12.4116659323139));
#35828=CARTESIAN_POINT('Ctrl Pts',(206.250989881508,5.39146815047745,-11.1950345470193));
#35829=CARTESIAN_POINT('Ctrl Pts',(206.369463033166,10.0714906457364,-7.27748607122799));
#35830=CARTESIAN_POINT('Ctrl Pts',(206.487936184825,12.3216625562562,-1.60416931544008));
#35831=CARTESIAN_POINT('Ctrl Pts',(206.606409336483,11.5991067909594,4.45616976693988));
#35832=CARTESIAN_POINT('Ctrl Pts',(206.724882488141,8.07814735173198,9.44141211399871));
#35833=CARTESIAN_POINT('Ctrl Pts',(206.8433556398,2.60825187482188,12.1488167941771));
#35834=CARTESIAN_POINT('Ctrl Pts',(206.961828791458,-3.49091116213162,11.9251946147582));
#35835=CARTESIAN_POINT('Ctrl Pts',(207.080301943116,-8.74785601816062,8.82449672372453));
#35836=CARTESIAN_POINT('Ctrl Pts',(207.198775094774,-11.8942907407006,3.5947983416629));
#35837=CARTESIAN_POINT('Ctrl Pts',(207.317248246433,-12.1711056287734,-2.50218207067393));
#35838=CARTESIAN_POINT('Ctrl Pts',(207.435721398091,-9.51151624683086,-7.99548535286034));
#35839=CARTESIAN_POINT('Ctrl Pts',(207.554194549749,-4.55717585595323,-11.5597956538802));
#35840=CARTESIAN_POINT('Ctrl Pts',(207.672667701408,1.49663002727809,-12.335186496482));
#35841=CARTESIAN_POINT('Ctrl Pts',(207.791140853066,7.18935854114184,-10.1345868740889));
#35842=CARTESIAN_POINT('Ctrl Pts',(207.909614004724,11.1475804487235,-5.48891405295993));
#35843=CARTESIAN_POINT('Ctrl Pts',(208.028087156383,12.4163340509309,0.481015672549472));
#35844=CARTESIAN_POINT('Ctrl Pts',(208.146560308041,10.6895195069813,6.33489542545181));
#35845=CARTESIAN_POINT('Ctrl Pts',(208.265033459699,6.38374856563713,10.6604165768637));
#35846=CARTESIAN_POINT('Ctrl Pts',(208.383506611358,0.537832700851228,12.4140027117541));
#35847=CARTESIAN_POINT('Ctrl Pts',(208.501979763016,-5.43784082831635,11.1725831600145));
#35848=CARTESIAN_POINT('Ctrl Pts',(208.620452914674,-10.1015793932378,7.23566314194201));
#35849=CARTESIAN_POINT('Ctrl Pts',(208.738926066333,-12.3282081532736,1.55306505694456));
#35850=CARTESIAN_POINT('Ctrl Pts',(208.857399217991,-11.5805300453036,-4.50422592809963));
#35851=CARTESIAN_POINT('Ctrl Pts',(208.975872369649,-8.03893009397561,-9.47482613485428));
#35852=CARTESIAN_POINT('Ctrl Pts',(209.094345521308,-2.55785567136515,-12.1595271991147));
#35853=CARTESIAN_POINT('Ctrl Pts',(209.212818672966,3.54032770950775,-11.9106174084653));
#35854=CARTESIAN_POINT('Ctrl Pts',(209.331291824624,8.78437065971439,-8.78814880701806));
#35855=CARTESIAN_POINT('Ctrl Pts',(209.449764976283,11.9090939440408,-3.54544902283972));
#35856=CARTESIAN_POINT('Ctrl Pts',(209.568238127941,12.1606259690128,2.55262676145886));
#35857=CARTESIAN_POINT('Ctrl Pts',(209.686711279599,9.47828204954912,8.03485511572791));
#35858=CARTESIAN_POINT('Ctrl Pts',(209.805184431257,4.50920521266752,11.5785921290801));
#35859=CARTESIAN_POINT('Ctrl Pts',(209.923657582916,-1.54776370605922,12.328874841272));
#35860=CARTESIAN_POINT('Ctrl Pts',(210.042130734574,-7.23131873010248,10.1046898401293));
#35861=CARTESIAN_POINT('Ctrl Pts',(210.160603886232,-11.1702438212084,5.44264460683406));
#35862=CARTESIAN_POINT('Ctrl Pts',(210.279077037891,-12.4142328355011,-0.532494551625294));
#35863=CARTESIAN_POINT('Ctrl Pts',(210.397550189549,-10.6631606434456,-6.37916392904402));
#35864=CARTESIAN_POINT('Ctrl Pts',(210.516023341207,-6.3394914006153,-10.6867944736983));
#35865=CARTESIAN_POINT('Ctrl Pts',(210.634496492866,-0.486354730070657,
-12.4161260632325));
#35866=CARTESIAN_POINT('Ctrl Pts',(210.752969644524,5.48412001555769,-11.1499396857787));
#35867=CARTESIAN_POINT('Ctrl Pts',(210.871442796182,10.1314944675793,-7.193715812774));
#35868=CARTESIAN_POINT('Ctrl Pts',(210.989915947841,12.3345417957047,-1.50193409694237));
#35869=CARTESIAN_POINT('Ctrl Pts',(211.108389099499,11.5617541995205,4.55220464955323));
#35870=CARTESIAN_POINT('Ctrl Pts',(211.226862251157,7.99957462566292,9.5080772583101));
#35871=CARTESIAN_POINT('Ctrl Pts',(211.345335402815,2.50741549156271,12.1700285494413));
#35872=CARTESIAN_POINT('Ctrl Pts',(211.463808554474,-3.58968338923699,11.8958354270131));
#35873=CARTESIAN_POINT('Ctrl Pts',(211.582281706132,-8.82073427459143,8.75164979867179));
#35874=CARTESIAN_POINT('Ctrl Pts',(211.700754857791,-11.9236923984033,3.49603874832707));
#35875=CARTESIAN_POINT('Ctrl Pts',(211.819228009449,-12.1499372357718,-2.60302756580651));
#35876=CARTESIAN_POINT('Ctrl Pts',(211.937701161107,-9.44488489540743,-8.07408673808059));
#35877=CARTESIAN_POINT('Ctrl Pts',(212.056174312765,-4.46115704415977,-11.5971895375081));
#35878=CARTESIAN_POINT('Ctrl Pts',(212.174647464424,1.59887077466865,-12.3223512199359));
#35879=CARTESIAN_POINT('Ctrl Pts',(212.293120616082,7.27315459347477,-10.0746190796953));
#35880=CARTESIAN_POINT('Ctrl Pts',(212.41159376774,11.1927151475138,-5.39628158718193));
#35881=CARTESIAN_POINT('Ctrl Pts',(212.530066919399,12.4119181864144,0.583964275704583));
#35882=CARTESIAN_POINT('Ctrl Pts',(212.648540071057,10.636618451838,6.42332275785386));
#35883=CARTESIAN_POINT('Ctrl Pts',(212.767013222715,6.29512524288724,10.7129886361327));
#35884=CARTESIAN_POINT('Ctrl Pts',(212.885486374374,0.434868397559615,12.4180359485044));
#35885=CARTESIAN_POINT('Ctrl Pts',(213.003959526032,-5.53030491620038,11.1271045144455));
#35886=CARTESIAN_POINT('Ctrl Pts',(213.12243267769,-10.1612353546035,7.15164480451173));
#35887=CARTESIAN_POINT('Ctrl Pts',(213.240905829348,-12.3406633745797,1.45077731470124));
#35888=CARTESIAN_POINT('Ctrl Pts',(213.359378981007,-11.542779576454,-4.60010510651003));
#35889=CARTESIAN_POINT('Ctrl Pts',(213.477852132665,-7.96008162340124,-9.5411649126474));
#35890=CARTESIAN_POINT('Ctrl Pts',(213.596325284324,-2.45693220262376,-12.1803206646317));
#35891=CARTESIAN_POINT('Ctrl Pts',(213.714798435982,3.63897735276813,-11.8808489245333));
#35892=CARTESIAN_POINT('Ctrl Pts',(213.83327158764,8.85694623760263,-8.71500032620544));
#35893=CARTESIAN_POINT('Ctrl Pts',(213.951744739299,11.9380858528027,-3.44656836761662));
#35894=CARTESIAN_POINT('Ctrl Pts',(214.070217890957,12.1390396128179,2.65338361719204));
#35895=CARTESIAN_POINT('Ctrl Pts',(214.188691042615,9.41132535859182,8.11317954542305));
#35896=CARTESIAN_POINT('Ctrl Pts',(214.307164194273,4.41303217650556,11.6155875594251));
#35897=CARTESIAN_POINT('Ctrl Pts',(214.425637345932,-1.64995035444002,12.315615744632));
#35898=CARTESIAN_POINT('Ctrl Pts',(214.54411049759,-7.31486541198911,10.0443751097831));
#35899=CARTESIAN_POINT('Ctrl Pts',(214.662583649248,-11.214994041298,5.3498257911071));
#35900=CARTESIAN_POINT('Ctrl Pts',(214.781056800907,-12.4093901434658,-0.635423959885912));
#35901=CARTESIAN_POINT('Ctrl Pts',(214.899529952565,-10.6098933884893,-6.46737115267362));
#35902=CARTESIAN_POINT('Ctrl Pts',(215.018003104223,-6.25065085522515,-10.7389986138195));
#35903=CARTESIAN_POINT('Ctrl Pts',(215.136476255882,-0.383374588505087,
-12.4197323347338));
#35904=CARTESIAN_POINT('Ctrl Pts',(215.25494940754,5.57639473620306,-11.1040780386123));
#35905=CARTESIAN_POINT('Ctrl Pts',(215.373422559198,10.1908015429855,-7.1094508404678));
#35906=CARTESIAN_POINT('Ctrl Pts',(215.491895710857,12.3465727846524,-1.39959558974226));
#35907=CARTESIAN_POINT('Ctrl Pts',(215.610368862515,11.5236065023283,4.64792647543395));
#35908=CARTESIAN_POINT('Ctrl Pts',(215.728842014173,7.92045176618019,9.57408852900145));
#35909=CARTESIAN_POINT('Ctrl Pts',(215.847315165832,2.40640667249019,12.1904033677372));
#35910=CARTESIAN_POINT('Ctrl Pts',(215.96578831749,-3.68820875260699,11.8656581586837));
#35911=CARTESIAN_POINT('Ctrl Pts',(216.084261469148,-8.8930059261681,8.67820101972081));
#35912=CARTESIAN_POINT('Ctrl Pts',(216.202734620806,-11.9522740597775,3.39703873123564));
#35913=CARTESIAN_POINT('Ctrl Pts',(216.321207772465,-12.1279332875099,-2.70369404986107));
#35914=CARTESIAN_POINT('Ctrl Pts',(216.439680924123,-9.37760401607995,-8.15213286564597));
#35915=CARTESIAN_POINT('Ctrl Pts',(216.558154075782,-4.36483143709935,-11.6337858785201));
#35916=CARTESIAN_POINT('Ctrl Pts',(216.67662722744,1.70100156717955,-12.3086685311612));
#35917=CARTESIAN_POINT('Ctrl Pts',(216.795100379098,7.35645046852558,-10.0139584503668));
#35918=CARTESIAN_POINT('Ctrl Pts',(216.913573530756,11.2370801195274,-5.30327801730832));
#35919=CARTESIAN_POINT('Ctrl Pts',(217.032046682415,12.4066487501191,0.686872719440438));
#35920=CARTESIAN_POINT('Ctrl Pts',(217.150519834073,10.5829859128744,6.51130835619429));
#35921=CARTESIAN_POINT('Ctrl Pts',(217.268992985731,6.20606900226191,10.7648239595782));
#35922=CARTESIAN_POINT('Ctrl Pts',(217.38746613739,0.331874188222308,12.4212151927553));
#35923=CARTESIAN_POINT('Ctrl Pts',(217.505939289048,-5.62238868315952,11.0808606541651));
#35924=CARTESIAN_POINT('Ctrl Pts',(217.624412440706,-10.220192524404,7.06713464606836));
#35925=CARTESIAN_POINT('Ctrl Pts',(217.742885592365,-12.3522699243242,1.3483898020152));
#35926=CARTESIAN_POINT('Ctrl Pts',(217.861358744023,-11.5042353067796,-4.69566793414851));
#35927=CARTESIAN_POINT('Ctrl Pts',(217.979831895681,-7.8806857353424,-9.60684754132778));
#35928=CARTESIAN_POINT('Ctrl Pts',(218.098305047339,-2.35583976983032,-12.2002764854091));
#35929=CARTESIAN_POINT('Ctrl Pts',(218.216778198998,3.73737674233492,-11.8502633906342));
#35930=CARTESIAN_POINT('Ctrl Pts',(218.335251350656,8.92891272032577,-8.64125251189527));
#35931=CARTESIAN_POINT('Ctrl Pts',(218.453724502314,11.9662567753948,-3.34745069073139));
#35932=CARTESIAN_POINT('Ctrl Pts',(218.572197653973,12.1166184507944,2.75395799884586));
#35933=CARTESIAN_POINT('Ctrl Pts',(218.690670805631,9.34372144763298,8.19094602903335));
#35934=CARTESIAN_POINT('Ctrl Pts',(218.80914395729,4.31655565463659,11.6517841819259));
#35935=CARTESIAN_POINT('Ctrl Pts',(218.927617108948,-1.75202353517421,12.301509698943));
#35936=CARTESIAN_POINT('Ctrl Pts',(219.046090260606,-7.39790904814131,9.98336962443466));
#35937=CARTESIAN_POINT('Ctrl Pts',(219.164563412264,-11.2589730024531,5.25663906597177));
#35938=CARTESIAN_POINT('Ctrl Pts',(219.283036563923,-12.4036940535703,-0.738309669631802));
#35939=CARTESIAN_POINT('Ctrl Pts',(219.401509715581,-10.5558964874704,-6.55513361342726));
#35940=CARTESIAN_POINT('Ctrl Pts',(219.519982867239,-6.16138045075807,-10.7904642285485));
#35941=CARTESIAN_POINT('Ctrl Pts',(219.638456018898,-0.28036808155549,-12.4224844988586));
#35942=CARTESIAN_POINT('Ctrl Pts',(219.756929170556,5.66828596508916,-11.0574527565455));
#35943=CARTESIAN_POINT('Ctrl Pts',(219.875402322214,10.2494077961033,-7.02469695662936));
#35944=CARTESIAN_POINT('Ctrl Pts',(219.993875473873,12.3577546903114,-1.29716081561161));
#35945=CARTESIAN_POINT('Ctrl Pts',(220.112348625531,11.4846663339971,4.74332862785197));
#35946=CARTESIAN_POINT('Ctrl Pts',(220.230821777189,7.84078419128066,9.6394414574504));
#35947=CARTESIAN_POINT('Ctrl Pts',(220.349294928848,2.30523241268773,12.2099396994737));
#35948=CARTESIAN_POINT('Ctrl Pts',(220.467768080506,-3.78648057830359,11.8346651951909));
#35949=CARTESIAN_POINT('Ctrl Pts',(220.586241232164,-8.96466579029084,8.60415478998313));
#35950=CARTESIAN_POINT('Ctrl Pts',(220.704714383822,-11.9800342031547,3.29780645257095));
#35951=CARTESIAN_POINT('Ctrl Pts',(220.823187535481,-12.1050943697152,-2.80417742887655));
#35952=CARTESIAN_POINT('Ctrl Pts',(220.941660687139,-9.30968017372072,-8.22961245759845));
#35953=CARTESIAN_POINT('Ctrl Pts',(221.060133838797,-4.26820161025575,-11.6695945107349));
#35954=CARTESIAN_POINT('Ctrl Pts',(221.178606990456,1.80300691838314,-12.2941135721597));
#35955=CARTESIAN_POINT('Ctrl Pts',(221.297080142114,7.43925808849352,-9.95266313161919));
#35956=CARTESIAN_POINT('Ctrl Pts',(221.415553293772,11.2806351168099,-5.20979760771178));
#35957=CARTESIAN_POINT('Ctrl Pts',(221.534026445431,12.4006004638457,0.789491960649636));
#35958=CARTESIAN_POINT('Ctrl Pts',(221.652499597089,10.5284385582057,6.59929565564178));
#35959=CARTESIAN_POINT('Ctrl Pts',(221.731481698195,7.58721771950252,9.40909253321683));
#35960=CARTESIAN_POINT('Ctrl Pts',(221.770972748747,5.87013955957299,10.380129409171));
#35961=CARTESIAN_POINT('Ctrl Pts',(220.768843152848,-11.9240373570162,-7.43698370121595E-5));
#35962=CARTESIAN_POINT('Ctrl Pts',(220.786957947059,-11.924234503617,-0.905127068583988));
#35963=CARTESIAN_POINT('Ctrl Pts',(220.80507274127,-11.8225000180031,-1.81013598156214));
#35964=CARTESIAN_POINT('Ctrl Pts',(220.823187535481,-11.6183486426227,-2.69141928675563));
#35965=CARTESIAN_POINT('Ctrl Pts',(220.862678586033,-11.1732896377171,-4.61265577178385));
#35966=CARTESIAN_POINT('Ctrl Pts',(220.902169636586,-10.2414849057189,-6.42113411469115));
#35967=CARTESIAN_POINT('Ctrl Pts',(220.941660687139,-8.93533611247564,-7.89870362833421));
#35968=CARTESIAN_POINT('Ctrl Pts',(220.981151737692,-7.6291873192324,-9.37627314197726));
#35969=CARTESIAN_POINT('Ctrl Pts',(221.020642788245,-5.94869446474407,-10.5229338263561));
#35970=CARTESIAN_POINT('Ctrl Pts',(221.060133838797,-4.09657994939343,-11.200350678783));
#35971=CARTESIAN_POINT('Ctrl Pts',(221.09962488935,-2.24446543404284,-11.8777675312098));
#35972=CARTESIAN_POINT('Ctrl Pts',(221.139115939903,-0.220729257829941,
-12.0859405516848));
#35973=CARTESIAN_POINT('Ctrl Pts',(221.178606990456,1.73051402529489,-11.7997853218322));
#35974=CARTESIAN_POINT('Ctrl Pts',(221.210737993637,3.31809914294103,-11.5669615688028));
#35975=CARTESIAN_POINT('Ctrl Pts',(221.242868996819,4.85769471604154,-11.0068976329263));
#35976=CARTESIAN_POINT('Ctrl Pts',(221.275,6.22722261202592,-10.1702729013571));
#35977=CARTESIAN_POINT('Ctrl Pts',(204.,-6.42465676560637,-9.01028147758817));
#35978=CARTESIAN_POINT('Ctrl Pts',(204.032131003181,-5.21120775505585,-9.87363627182968));
#35979=CARTESIAN_POINT('Ctrl Pts',(204.103753056916,-2.11541440506495,-11.252056127613));
#35980=CARTESIAN_POINT('Ctrl Pts',(204.214866161202,3.19351689060185,-11.0794786062488));
#35981=CARTESIAN_POINT('Ctrl Pts',(204.333339312861,8.08365868074054,-8.22238332192522));
#35982=CARTESIAN_POINT('Ctrl Pts',(204.451812464519,11.0235253467705,-3.38157672049597));
#35983=CARTESIAN_POINT('Ctrl Pts',(204.570285616177,11.303857784602,2.27508107448027));
#35984=CARTESIAN_POINT('Ctrl Pts',(204.688758767836,8.85701624610765,7.38284688961676));
#35985=CARTESIAN_POINT('Ctrl Pts',(204.807231919494,4.27332958062524,10.7094275823243));
#35986=CARTESIAN_POINT('Ctrl Pts',(204.925705071152,-1.34134224161475,11.4522476363554));
#35987=CARTESIAN_POINT('Ctrl Pts',(205.044178222811,-6.63240123149158,9.43209587689214));
#35988=CARTESIAN_POINT('Ctrl Pts',(205.15990000046,-10.2376088257201,5.23611643961605));
#35989=CARTESIAN_POINT('Ctrl Pts',(205.236130727557,-11.0657697006446,1.70247381065806));
#35990=CARTESIAN_POINT('Ctrl Pts',(205.272870404101,-11.066766136903,-0.000127008754821131));
#35991=CARTESIAN_POINT('Origin',(201.227129595899,0.,0.));
#35992=CARTESIAN_POINT('Ctrl Pts',(204.,6.42428395783811,-9.01020671414169));
#35993=CARTESIAN_POINT('Ctrl Pts',(204.039491050553,7.91474988128163,-7.9475034238105));
#35994=CARTESIAN_POINT('Ctrl Pts',(204.118473151658,10.3565945407743,-5.06910807865537));
#35995=CARTESIAN_POINT('Ctrl Pts',(204.236946303317,11.5208305663343,0.474233997127887));
#35996=CARTESIAN_POINT('Ctrl Pts',(204.355419454975,9.90531651320884,5.90221595067179));
#35997=CARTESIAN_POINT('Ctrl Pts',(204.473892606633,5.90014038006902,9.90669837751048));
#35998=CARTESIAN_POINT('Ctrl Pts',(204.592365758292,0.471446650502101,11.5208655173499));
#35999=CARTESIAN_POINT('Ctrl Pts',(204.71083890995,-5.07096553594642,10.3556122261992));
#36000=CARTESIAN_POINT('Ctrl Pts',(204.829312061608,-9.38996616253539,6.69191003627886));
#36001=CARTESIAN_POINT('Ctrl Pts',(204.918075623591,-10.9285607524451,2.73735033409805));
#36002=CARTESIAN_POINT('Ctrl Pts',(204.967348135022,-11.0663132288553,0.45368304064905));
#36003=CARTESIAN_POINT('Ctrl Pts',(204.977129595899,-11.0658620952239,0.000280741946515339));
#36004=CARTESIAN_POINT('Ctrl Pts',(203.504027251253,6.92300129651942,-9.70966930685028));
#36005=CARTESIAN_POINT('Ctrl Pts',(203.543518301805,8.52917213020871,-8.56446833113655));
#36006=CARTESIAN_POINT('Ctrl Pts',(203.622500402911,11.1605772571476,-5.46262307691302));
#36007=CARTESIAN_POINT('Ctrl Pts',(203.740973554569,12.4151929570924,0.511048795245736));
#36008=CARTESIAN_POINT('Ctrl Pts',(203.859446706228,10.6742665040069,6.36040513573264));
#36009=CARTESIAN_POINT('Ctrl Pts',(203.977919857886,6.35816843852751,10.6757556424719));
#36010=CARTESIAN_POINT('Ctrl Pts',(204.096393009544,0.508045066825541,12.4152306213563));
#36011=CARTESIAN_POINT('Ctrl Pts',(204.214866161202,-5.46462472866412,11.1595186854654));
#36012=CARTESIAN_POINT('Ctrl Pts',(204.333339312861,-10.1189094915696,7.21140319472127));
#36013=CARTESIAN_POINT('Ctrl Pts',(204.451812464519,-12.3318977278251,1.52348893979719));
#36014=CARTESIAN_POINT('Ctrl Pts',(204.570285616177,-11.5696916564292,-4.53199528109509));
#36015=CARTESIAN_POINT('Ctrl Pts',(204.688758767836,-8.01617731810691,-9.49408304713466));
#36016=CARTESIAN_POINT('Ctrl Pts',(204.807231919494,-2.52867846986942,-12.1656286313568));
#36017=CARTESIAN_POINT('Ctrl Pts',(204.925705071153,3.56889033400025,-11.9020899448289));
#36018=CARTESIAN_POINT('Ctrl Pts',(205.044178222811,8.80542753846537,-8.76705044750802));
#36019=CARTESIAN_POINT('Ctrl Pts',(205.162651374469,11.9175649567678,-3.51686964666669));
#36020=CARTESIAN_POINT('Ctrl Pts',(205.281124526127,12.1544673643034,2.58179193456698));
#36021=CARTESIAN_POINT('Ctrl Pts',(205.399597677786,9.45897966964662,8.05756976071132));
#36022=CARTESIAN_POINT('Ctrl Pts',(205.518070829444,4.48141594756073,11.5893760697451));
#36023=CARTESIAN_POINT('Ctrl Pts',(205.636543981102,-1.57733540710525,12.325126357774));
#36024=CARTESIAN_POINT('Ctrl Pts',(205.755017132761,-7.25553839212175,10.0873132846628));
#36025=CARTESIAN_POINT('Ctrl Pts',(205.873490284419,-11.1832682011054,5.41583225572877));
#36026=CARTESIAN_POINT('Ctrl Pts',(205.991963436077,-12.4129196682143,-0.562273945038027));
#36027=CARTESIAN_POINT('Ctrl Pts',(206.110436587736,-10.647826743886,-6.40472577929877));
#36028=CARTESIAN_POINT('Ctrl Pts',(206.228909739394,-6.31383622967067,-10.7019717222351));
#36029=CARTESIAN_POINT('Ctrl Pts',(206.347382891052,-0.456567861250994,
-12.4172570427219));
#36030=CARTESIAN_POINT('Ctrl Pts',(206.46585604271,5.51085219412049,-11.1367515358957));
#36031=CARTESIAN_POINT('Ctrl Pts',(206.584329194369,10.1487225431899,-7.16939031011746));
#36032=CARTESIAN_POINT('Ctrl Pts',(206.702802346027,12.3381093181286,-1.4723400189527));
#36033=CARTESIAN_POINT('Ctrl Pts',(206.821275497686,11.5508004673251,4.57992742754356));
#36034=CARTESIAN_POINT('Ctrl Pts',(206.939748649344,7.97674233926988,9.52724033130231));
#36035=CARTESIAN_POINT('Ctrl Pts',(207.058221801002,2.47821317462715,12.1760086292109));
#36036=CARTESIAN_POINT('Ctrl Pts',(207.17669495266,-3.61821037775123,11.8871897578796));
#36037=CARTESIAN_POINT('Ctrl Pts',(207.295168104319,-8.84170350563972,8.73046423713344));
#36038=CARTESIAN_POINT('Ctrl Pts',(207.413641255977,-11.9320448295726,3.46742452874975));
#36039=CARTESIAN_POINT('Ctrl Pts',(207.532114407635,-12.1436577572359,-2.63216696898803));
#36040=CARTESIAN_POINT('Ctrl Pts',(207.650587559294,-9.42548849587364,-8.09672114449177));
#36041=CARTESIAN_POINT('Ctrl Pts',(207.769060710952,-4.43332330428022,-11.6078581640728));
#36042=CARTESIAN_POINT('Ctrl Pts',(207.88753386261,1.62842667920446,-12.3184801508937));
#36043=CARTESIAN_POINT('Ctrl Pts',(208.006007014269,7.29730199706176,-10.0571422502212));
#36044=CARTESIAN_POINT('Ctrl Pts',(208.124480165927,11.2056282409638,-5.36941546193074));
#36045=CARTESIAN_POINT('Ctrl Pts',(208.242953317585,12.4104815532728,0.613737968013001));
#36046=CARTESIAN_POINT('Ctrl Pts',(208.361426469244,10.6211786946092,6.44882080807686));
#36047=CARTESIAN_POINT('Ctrl Pts',(208.479899620902,6.26940736161951,10.7280593777056));
#36048=CARTESIAN_POINT('Ctrl Pts',(208.59837277256,0.405077095315529,12.419043410197));
#36049=CARTESIAN_POINT('Ctrl Pts',(208.716845924218,-5.55698218170029,11.1138056357744));
#36050=CARTESIAN_POINT('Ctrl Pts',(208.835319075877,-10.1783624189946,7.12724807657941));
#36051=CARTESIAN_POINT('Ctrl Pts',(208.953792227535,-12.3441081576266,1.42116869875556));
#36052=CARTESIAN_POINT('Ctrl Pts',(209.072265379193,-11.5317109888576,-4.6277822276949));
#36053=CARTESIAN_POINT('Ctrl Pts',(209.190738530852,-7.93717007562952,-9.560233149251));
#36054=CARTESIAN_POINT('Ctrl Pts',(209.30921168251,-2.42770534095333,-12.1861796086802));
#36055=CARTESIAN_POINT('Ctrl Pts',(209.427684834168,3.66746824770378,-11.8720850455845));
#36056=CARTESIAN_POINT('Ctrl Pts',(209.546157985827,8.87782744470561,-8.69372800008941));
#36057=CARTESIAN_POINT('Ctrl Pts',(209.664631137485,11.9463195663411,-3.41791976154524));
#36058=CARTESIAN_POINT('Ctrl Pts',(209.783104289143,12.1326393648134,2.68249673268913));
#36059=CARTESIAN_POINT('Ctrl Pts',(209.901577440802,9.391835274627,8.1357333321452));
#36060=CARTESIAN_POINT('Ctrl Pts',(210.02005059246,4.38515443956386,11.6261406846245));
#36061=CARTESIAN_POINT('Ctrl Pts',(210.138523744118,-1.6794899539259,12.3116221584391));
#36062=CARTESIAN_POINT('Ctrl Pts',(210.256996895776,-7.33894014217483,10.0267983058941));
#36063=CARTESIAN_POINT('Ctrl Pts',(210.375470047435,-11.2277956262,5.32290635403163));
#36064=CARTESIAN_POINT('Ctrl Pts',(210.493943199093,-12.4078300692124,-0.665191439402797));
#36065=CARTESIAN_POINT('Ctrl Pts',(210.612416350752,-10.5943480390211,-6.49280496438909));
#36066=CARTESIAN_POINT('Ctrl Pts',(210.73088950241,-6.22487070580297,-10.7539625893687));
#36067=CARTESIAN_POINT('Ctrl Pts',(210.849362654068,-0.353579365023488,
-12.4206162612866));
#36068=CARTESIAN_POINT('Ctrl Pts',(210.967835805727,5.60301662998475,-11.0906686598068));
#36069=CARTESIAN_POINT('Ctrl Pts',(211.086308957385,10.2078273016985,-7.08498330669916));
#36070=CARTESIAN_POINT('Ctrl Pts',(211.204782109043,12.3498947690968,-1.36997294489374));
#36071=CARTESIAN_POINT('Ctrl Pts',(211.323255260701,11.5124232496295,4.67555746397121));
#36072=CARTESIAN_POINT('Ctrl Pts',(211.44172841236,7.89746135094013,9.59306160138219));
#36073=CARTESIAN_POINT('Ctrl Pts',(211.560201564018,2.37715576857242,12.196141075334));
#36074=CARTESIAN_POINT('Ctrl Pts',(211.678674715676,-3.71666306412984,11.8567762205938));
#36075=CARTESIAN_POINT('Ctrl Pts',(211.797147867335,-8.91379875032231,8.65684229475499));
#36076=CARTESIAN_POINT('Ctrl Pts',(211.915621018993,-11.9603889141255,3.36835623121586));
#36077=CARTESIAN_POINT('Ctrl Pts',(212.034094170651,-12.1214123800741,-2.7327803771419));
#36078=CARTESIAN_POINT('Ctrl Pts',(212.15256732231,-9.35802058277042,-8.17460564491962));
#36079=CARTESIAN_POINT('Ctrl Pts',(212.271040473968,-4.33691018238782,-11.6442233209179));
#36080=CARTESIAN_POINT('Ctrl Pts',(212.389513625626,1.73052435375133,-12.3045524964779));
#36081=CARTESIAN_POINT('Ctrl Pts',(212.507986777285,7.38045211140153,-9.99628197425497));
#36082=CARTESIAN_POINT('Ctrl Pts',(212.626459928943,11.2497699757883,-5.27630573122507));
#36083=CARTESIAN_POINT('Ctrl Pts',(212.744933080601,12.4049652615757,0.716633474383855));
#36084=CARTESIAN_POINT('Ctrl Pts',(212.86340623226,10.5673352384327,6.53667749212747));
#36085=CARTESIAN_POINT('Ctrl Pts',(212.981879383918,6.18022702791458,10.7796809118332));
#36086=CARTESIAN_POINT('Ctrl Pts',(213.100352535576,0.302075555762362,12.4219755689712));
#36087=CARTESIAN_POINT('Ctrl Pts',(213.218825687234,-5.64895474752174,11.0673410057682));
#36088=CARTESIAN_POINT('Ctrl Pts',(213.337298838893,-10.2371166847208,7.04259672712543));
#36089=CARTESIAN_POINT('Ctrl Pts',(213.455771990551,-12.3554690530526,1.31875363755592));
#36090=CARTESIAN_POINT('Ctrl Pts',(213.57424514221,-11.4929375812482,-4.72325231498802));
#36091=CARTESIAN_POINT('Ctrl Pts',(213.692718293868,-7.85761684790037,-9.62572512328807));
#36092=CARTESIAN_POINT('Ctrl Pts',(213.811191445526,-2.32656532656588,-12.2058928579079));
#36093=CARTESIAN_POINT('Ctrl Pts',(213.929664597184,3.76579398123967,-11.8412635461071));
#36094=CARTESIAN_POINT('Ctrl Pts',(214.048137748843,8.94961680404746,-8.6198077552935));
#36095=CARTESIAN_POINT('Ctrl Pts',(214.166610900501,11.9742526310362,-3.31873478989055));
#36096=CARTESIAN_POINT('Ctrl Pts',(214.285084052159,12.1099769960399,2.78301703783682));
#36097=CARTESIAN_POINT('Ctrl Pts',(214.403557203818,9.32404500166837,8.21333741449657));
#36098=CARTESIAN_POINT('Ctrl Pts',(214.522030355476,4.2885913621992,11.6621057620645));
#36099=CARTESIAN_POINT('Ctrl Pts',(214.640503507134,-1.78152900126369,12.2972712865563));
#36100=CARTESIAN_POINT('Ctrl Pts',(214.758976658793,-7.42183719104071,9.9655937799607));
#36101=CARTESIAN_POINT('Ctrl Pts',(214.877449810451,-11.2715509119312,5.22961439469969));
#36102=CARTESIAN_POINT('Ctrl Pts',(214.995922962109,-12.4018871796163,-0.768063188530766));
#36103=CARTESIAN_POINT('Ctrl Pts',(215.114396113768,-10.5401407572657,-6.58043763700659));
#36104=CARTESIAN_POINT('Ctrl Pts',(215.232869265426,-6.13547709549785,-10.8052139029326));
#36105=CARTESIAN_POINT('Ctrl Pts',(215.351342417084,-0.25056655301961,-12.4231213098808));
#36106=CARTESIAN_POINT('Ctrl Pts',(215.469815568742,5.69479574451283,-11.043823074723));
#36107=CARTESIAN_POINT('Ctrl Pts',(215.588288720401,10.2662300644991,-7.00008906659626));
#36108=CARTESIAN_POINT('Ctrl Pts',(215.706761872059,12.360830913657,-1.2675116573381));
#36109=CARTESIAN_POINT('Ctrl Pts',(215.825235023717,11.473254318724,4.77086596074414));
#36110=CARTESIAN_POINT('Ctrl Pts',(215.943708175376,7.81763725154309,9.65822315339587));
#36111=CARTESIAN_POINT('Ctrl Pts',(216.062181327034,2.27593488471799,12.2154347887429));
#36112=CARTESIAN_POINT('Ctrl Pts',(216.180654478692,-3.8148601543422,11.8255472888285));
#36113=CARTESIAN_POINT('Ctrl Pts',(216.299127630351,-8.98528099007356,8.58262501842705));
#36114=CARTESIAN_POINT('Ctrl Pts',(216.417600782009,-11.9879104787191,3.2690562906936));
#36115=CARTESIAN_POINT('Ctrl Pts',(216.536073933667,-12.0983334093154,-2.83320585107222));
#36116=CARTESIAN_POINT('Ctrl Pts',(216.654547085326,-9.28990911545137,-8.25192797497408));
#36117=CARTESIAN_POINT('Ctrl Pts',(216.773020236984,-4.24019880972685,-11.6797877006176));
#36118=CARTESIAN_POINT('Ctrl Pts',(216.891493388642,1.83250301955755,-12.2897786538578));
#36119=CARTESIAN_POINT('Ctrl Pts',(217.009966540301,7.46309466957279,-9.93473425062294));
#36120=CARTESIAN_POINT('Ctrl Pts',(217.128439691959,11.2931380601564,-5.18283314720375));
#36121=CARTESIAN_POINT('Ctrl Pts',(217.246912843617,12.3985958762547,0.819479697630158));
#36122=CARTESIAN_POINT('Ctrl Pts',(217.365385995275,10.5127650630656,6.62408464667336));
#36123=CARTESIAN_POINT('Ctrl Pts',(217.483859146934,6.09062167792295,10.8305611236871));
#36124=CARTESIAN_POINT('Ctrl Pts',(217.602332298592,0.199053242371885,12.4240534643169));
#36125=CARTESIAN_POINT('Ctrl Pts',(217.720805450251,-5.74053883282964,11.0201152710073));
#36126=CARTESIAN_POINT('Ctrl Pts',(217.839278601909,-10.2951669404969,6.95746105593078));
#36127=CARTESIAN_POINT('Ctrl Pts',(217.957751753567,-12.3659802587261,1.21624788522728));
#36128=CARTESIAN_POINT('Ctrl Pts',(218.076224905225,-11.4533738004635,-4.81839758263655));
#36129=CARTESIAN_POINT('Ctrl Pts',(218.194698056884,-7.77752324922622,-9.69055513297366));
#36130=CARTESIAN_POINT('Ctrl Pts',(218.313171208542,-2.2252653134951,-12.2247667037974));
#36131=CARTESIAN_POINT('Ctrl Pts',(218.4316443602,3.86386073984913,-11.8096277189421));
#36132=CARTESIAN_POINT('Ctrl Pts',(218.550117511859,9.02079069526072,-8.54529472346733));
#36133=CARTESIAN_POINT('Ctrl Pts',(218.668590663517,12.0013622223129,-3.2193215876436));
#36134=CARTESIAN_POINT('Ctrl Pts',(218.787063815175,12.086481820182,2.88334595378683));
#36135=CARTESIAN_POINT('Ctrl Pts',(218.905536966834,9.25561351080288,8.29037666325784));
#36136=CARTESIAN_POINT('Ctrl Pts',(219.024010118492,4.19173335739202,11.6972688317836));
#36137=CARTESIAN_POINT('Ctrl Pts',(219.14248327015,-1.88344553314147,12.2820747288597));
#36138=CARTESIAN_POINT('Ctrl Pts',(219.260956421808,-7.50422383581897,9.90370391333251));
#36139=CARTESIAN_POINT('Ctrl Pts',(219.379429573467,-11.3145310531959,5.13596280027263));
#36140=CARTESIAN_POINT('Ctrl Pts',(219.497902725125,-12.3950913999872,-0.870882132825059));
#36141=CARTESIAN_POINT('Ctrl Pts',(219.616375876784,-10.4852086433947,-6.66761773911089));
#36142=CARTESIAN_POINT('Ctrl Pts',(219.734849028442,-6.04566151106375,-10.8557222043472));
#36143=CARTESIAN_POINT('Ctrl Pts',(219.8533221801,-0.147536583240307,-12.4247718782891));
#36144=CARTESIAN_POINT('Ctrl Pts',(219.971795331759,5.78618338014802,-10.9962182904565));
#36145=CARTESIAN_POINT('Ctrl Pts',(220.090268483417,10.3239264932221,-6.91471282583509));
#36146=CARTESIAN_POINT('Ctrl Pts',(220.208741635075,12.3709176724325,-1.16496446066495));
#36147=CARTESIAN_POINT('Ctrl Pts',(220.327214786733,11.4332949628521,4.86584899186587));
#36148=CARTESIAN_POINT('Ctrl Pts',(220.445687938392,7.73727846682914,9.72271501496135));
#36149=CARTESIAN_POINT('Ctrl Pts',(220.56416109005,2.17455134987996,12.2338999155263));
#36150=CARTESIAN_POINT('Ctrl Pts',(220.682634241708,-3.91278207789302,11.7934811477489));
#36151=CARTESIAN_POINT('Ctrl Pts',(220.801107393367,-9.05617206812273,8.50786764724348));
#36152=CARTESIAN_POINT('Ctrl Pts',(220.919580545025,-12.0145515263405,3.16942747355545));
#36153=CARTESIAN_POINT('Ctrl Pts',(221.038053696683,-12.0745376864656,-2.9332109864585));
#36154=CARTESIAN_POINT('Ctrl Pts',(221.156526848342,-9.22089667210347,-8.32909359747953));
#36155=CARTESIAN_POINT('Ctrl Pts',(221.235508949447,-5.83600017639687,-10.5848002797816));
#36156=CARTESIAN_POINT('Ctrl Pts',(221.275,-3.97626028075542,-11.2425521648639));
#36157=CARTESIAN_POINT('Ctrl Pts',(203.669351500835,6.75676218362565,-9.47651510928075));
#36158=CARTESIAN_POINT('Ctrl Pts',(203.708842551388,8.32436471389968,-8.35881336202787));
#36159=CARTESIAN_POINT('Ctrl Pts',(203.787824652493,10.8925830183565,-5.33145141082714));
#36160=CARTESIAN_POINT('Ctrl Pts',(203.906297804152,12.117072160173,0.498777195873124));
#36161=CARTESIAN_POINT('Ctrl Pts',(204.02477095581,10.4179498404076,6.20767540737902));
#36162=CARTESIAN_POINT('Ctrl Pts',(204.143244107468,6.20549241904135,10.4194032208181));
#36163=CARTESIAN_POINT('Ctrl Pts',(204.261717259127,0.495845594717724,12.1171089200209));
#36164=CARTESIAN_POINT('Ctrl Pts',(204.380190410785,-5.33340499775821,10.89154986571));
#36165=CARTESIAN_POINT('Ctrl Pts',(204.498663562443,-9.87592838189151,7.0382388085738));
#36166=CARTESIAN_POINT('Ctrl Pts',(204.617136714102,-12.0357770641469,1.48690604185916));
#36167=CARTESIAN_POINT('Ctrl Pts',(204.73560986576,-11.2918735259622,-4.42317038811887));
#36168=CARTESIAN_POINT('Ctrl Pts',(204.854083017418,-7.82368823005323,-9.26610563157517));
#36169=CARTESIAN_POINT('Ctrl Pts',(204.972556169076,-2.46795837931619,-11.873500517429));
#36170=CARTESIAN_POINT('Ctrl Pts',(205.091029320735,3.48319207428195,-11.6162900743298));
#36171=CARTESIAN_POINT('Ctrl Pts',(205.209502472393,8.59398651744738,-8.5565309594037));
#36172=CARTESIAN_POINT('Ctrl Pts',(205.327975624052,11.6313934913279,-3.43242053779264));
#36173=CARTESIAN_POINT('Ctrl Pts',(205.44644877571,11.8626072611781,2.51979645276714));
#36174=CARTESIAN_POINT('Ctrl Pts',(205.564921927368,9.23184517669876,7.86408673337551));
#36175=CARTESIAN_POINT('Ctrl Pts',(205.683395079026,4.37380559480734,11.3110852657559));
#36176=CARTESIAN_POINT('Ctrl Pts',(205.801868230685,-1.53945951663779,12.0291682921515));
#36177=CARTESIAN_POINT('Ctrl Pts',(205.920341382343,-7.08131420607698,9.84509088138708));
#36178=CARTESIAN_POINT('Ctrl Pts',(206.038814534001,-10.9147290942386,5.28578415791509));
#36179=CARTESIAN_POINT('Ctrl Pts',(206.15728768566,-12.1148534588228,-0.548772297728888));
#36180=CARTESIAN_POINT('Ctrl Pts',(206.275760837318,-10.3921449671051,-6.2509317980072));
#36181=CARTESIAN_POINT('Ctrl Pts',(206.394233988976,-6.16222474083492,-10.4449897849049));
#36182=CARTESIAN_POINT('Ctrl Pts',(206.512707140635,-0.44560448958899,-12.119086681784));
#36183=CARTESIAN_POINT('Ctrl Pts',(206.631180292293,5.37852242256608,-10.8693294141092));
#36184=CARTESIAN_POINT('Ctrl Pts',(206.749653443951,9.90502554526596,-6.99723476166445));
#36185=CARTESIAN_POINT('Ctrl Pts',(206.868126595609,12.0418394981499,-1.43698533849758));
#36186=CARTESIAN_POINT('Ctrl Pts',(206.986599747268,11.2734359630216,4.4699515601325));
#36187=CARTESIAN_POINT('Ctrl Pts',(207.105072898926,7.78520018674576,9.29846672385004));
#36188=CARTESIAN_POINT('Ctrl Pts',(207.223546050585,2.41870488594333,11.8836312647686));
#36189=CARTESIAN_POINT('Ctrl Pts',(207.342019202243,-3.53132781660499,11.601747679291));
#36190=CARTESIAN_POINT('Ctrl Pts',(207.460492353901,-8.62939140510808,8.52082327828202));
#36191=CARTESIAN_POINT('Ctrl Pts',(207.578965505559,-11.6455256650487,3.38416272465686));
#36192=CARTESIAN_POINT('Ctrl Pts',(207.697438657218,-11.8520572206502,-2.56896185271385));
#36193=CARTESIAN_POINT('Ctrl Pts',(207.815911808876,-9.19915821236894,-7.902297991475));
#36194=CARTESIAN_POINT('Ctrl Pts',(207.934384960534,-4.32686777990447,-11.3291235573406));
#36195=CARTESIAN_POINT('Ctrl Pts',(208.052858112193,1.5893239555491,-12.0226816778364));
#36196=CARTESIAN_POINT('Ctrl Pts',(208.171331263851,7.12207495917007,-9.81564433128193));
#36197=CARTESIAN_POINT('Ctrl Pts',(208.28980441551,10.9365522118821,-5.24048195102726));
#36198=CARTESIAN_POINT('Ctrl Pts',(208.408277567168,12.1124738893081,0.599000536806266));
#36199=CARTESIAN_POINT('Ctrl Pts',(208.526750718826,10.3661368062066,6.29396799144016));
#36200=CARTESIAN_POINT('Ctrl Pts',(208.645223870484,6.11886272447068,10.4704510084976));
#36201=CARTESIAN_POINT('Ctrl Pts',(208.763697022143,0.395350149718566,12.1208301539697));
#36202=CARTESIAN_POINT('Ctrl Pts',(208.882170173801,-5.42354471019256,10.8469345042186));
#36203=CARTESIAN_POINT('Ctrl Pts',(209.000643325459,-9.93395369122276,6.95610447182229));
#36204=CARTESIAN_POINT('Ctrl Pts',(209.119116477118,-12.0476942900429,1.38704277364959));
#36205=CARTESIAN_POINT('Ctrl Pts',(209.237589628776,-11.2548048721566,-4.51665724313303));
#36206=CARTESIAN_POINT('Ctrl Pts',(209.356062780434,-7.7465781551971,-9.33066729916396));
#36207=CARTESIAN_POINT('Ctrl Pts',(209.474535932092,-2.36940987559633,-11.8935580127938));
#36208=CARTESIAN_POINT('Ctrl Pts',(209.593009083751,3.57940287808283,-11.5870056700874));
#36209=CARTESIAN_POINT('Ctrl Pts',(209.711482235409,8.66464791524722,-8.48496917301807));
#36210=CARTESIAN_POINT('Ctrl Pts',(209.829955387067,11.6594576285783,-3.33584669456673));
#36211=CARTESIAN_POINT('Ctrl Pts',(209.948428538726,11.8413034082419,2.61808306900733));
#36212=CARTESIAN_POINT('Ctrl Pts',(210.066901690384,9.16631309174318,7.9403733959054));
#36213=CARTESIAN_POINT('Ctrl Pts',(210.185374842042,4.27985557383898,11.3469670674301));
#36214=CARTESIAN_POINT('Ctrl Pts',(210.303847993701,-1.63916106937189,12.0159883634648));
#36215=CARTESIAN_POINT('Ctrl Pts',(210.422321145359,-7.16271326505017,9.78602902330351));
#36216=CARTESIAN_POINT('Ctrl Pts',(210.540794297018,-10.9581873010376,5.19508964673795));
#36217=CARTESIAN_POINT('Ctrl Pts',(210.659267448676,-12.1098860742171,-0.649218477669228));
#36218=CARTESIAN_POINT('Ctrl Pts',(210.777740600334,-10.3399504238451,-6.33689597474106));
#36219=CARTESIAN_POINT('Ctrl Pts',(210.896213751992,-6.07539550860324,-10.4957322172542));
#36220=CARTESIAN_POINT('Ctrl Pts',(211.014686903651,-0.345089012723726,
-12.1223652368489));
#36221=CARTESIAN_POINT('Ctrl Pts',(211.133160055309,5.46847375266852,-10.8243531067053));
#36222=CARTESIAN_POINT('Ctrl Pts',(211.251633206967,9.96271104611431,-6.9148545880515));
#36223=CARTESIAN_POINT('Ctrl Pts',(211.370106358626,12.0533419500502,-1.33707636185219));
#36224=CARTESIAN_POINT('Ctrl Pts',(211.488579510284,11.235980281283,4.56328527279234));
#36225=CARTESIAN_POINT('Ctrl Pts',(211.607052661942,7.70782293938106,9.3627074555075));
#36226=CARTESIAN_POINT('Ctrl Pts',(211.7255258136,2.32007412879624,11.9032802789464));
#36227=CARTESIAN_POINT('Ctrl Pts',(211.843998965259,-3.62741640011194,11.5720644494603));
#36228=CARTESIAN_POINT('Ctrl Pts',(211.962472116917,-8.69975545705987,8.44896918858282));
#36229=CARTESIAN_POINT('Ctrl Pts',(212.080945268576,-11.6731891350429,3.2874733124059));
#36230=CARTESIAN_POINT('Ctrl Pts',(212.199418420234,-11.8303460123564,-2.66715927349457));
#36231=CARTESIAN_POINT('Ctrl Pts',(212.317891571892,-9.1333103778332,-7.97831228421332));
#36232=CARTESIAN_POINT('Ctrl Pts',(212.43636472355,-4.23276978568116,-11.364615492998));
#36233=CARTESIAN_POINT('Ctrl Pts',(212.554837875209,1.68897000165938,-12.0090884623172));
#36234=CARTESIAN_POINT('Ctrl Pts',(212.673311026867,7.20322842485229,-9.75624546747695));
#36235=CARTESIAN_POINT('Ctrl Pts',(212.791784178525,10.9796339898288,-5.1496080250501));
#36236=CARTESIAN_POINT('Ctrl Pts',(212.910257330184,12.107090057999,0.699425256741116));
#36237=CARTESIAN_POINT('Ctrl Pts',(213.028730481842,10.3135862702544,6.37971500995803));
#36238=CARTESIAN_POINT('Ctrl Pts',(213.1472036335,6.03182384053987,10.5208329764786));
#36239=CARTESIAN_POINT('Ctrl Pts',(213.265676785159,0.294821942731522,12.1236919040509));
#36240=CARTESIAN_POINT('Ctrl Pts',(213.384149936817,-5.51330877754666,10.8015856097932));
#36241=CARTESIAN_POINT('Ctrl Pts',(213.502623088475,-9.99129711552418,6.87348581955205));
#36242=CARTESIAN_POINT('Ctrl Pts',(213.621096240133,-12.0587823810742,1.2870869621585));
#36243=CARTESIAN_POINT('Ctrl Pts',(213.739569391792,-11.2169625140456,-4.60983484744952));
#36244=CARTESIAN_POINT('Ctrl Pts',(213.85804254345,-7.66893520560297,-9.39458664202572));
#36245=CARTESIAN_POINT('Ctrl Pts',(213.976515695109,-2.27069849375563,-11.9127978960747));
#36246=CARTESIAN_POINT('Ctrl Pts',(214.094988846767,3.67536755721219,-11.5569242742893));
#36247=CARTESIAN_POINT('Ctrl Pts',(214.213461998425,8.73471342695404,-8.41282394391167));
#36248=CARTESIAN_POINT('Ctrl Pts',(214.331935150083,11.6867199483614,-3.23904340984146));
#36249=CARTESIAN_POINT('Ctrl Pts',(214.450408301742,11.8191852213803,2.71618962242513));
#36250=CARTESIAN_POINT('Ctrl Pts',(214.5688814534,9.10015063804339,8.01611400412836));
#36251=CARTESIAN_POINT('Ctrl Pts',(214.687354605058,4.18561122496097,11.3820685306207));
#36252=CARTESIAN_POINT('Ctrl Pts',(214.805827756717,-1.73874989606355,12.0019820930213));
#36253=CARTESIAN_POINT('Ctrl Pts',(214.924300908375,-7.24361974201309,9.72629417586076));
#36254=CARTESIAN_POINT('Ctrl Pts',(215.042774060033,-11.0008919095302,5.10403786791374));
#36255=CARTESIAN_POINT('Ctrl Pts',(215.161247211692,-12.1040858887246,-0.749620010833857));
#36256=CARTESIAN_POINT('Ctrl Pts',(215.27972036335,-10.2870447987044,-6.42242436091798));
#36257=CARTESIAN_POINT('Ctrl Pts',(215.398193515008,-5.98814846939336,-10.5457528546219));
#36258=CARTESIAN_POINT('Ctrl Pts',(215.516666666667,-0.244549803966582,
-12.1248101327668));
#36259=CARTESIAN_POINT('Ctrl Pts',(215.635139818325,5.55804901399366,-10.7786324049162));
#36260=CARTESIAN_POINT('Ctrl Pts',(215.753612969983,10.0197114079818,-6.83199887756314));
#36261=CARTESIAN_POINT('Ctrl Pts',(215.872086121641,12.0640154895794,-1.23707543401911));
#36262=CARTESIAN_POINT('Ctrl Pts',(215.9905592733,11.1977518974102,4.6563051667937));
#36263=CARTESIAN_POINT('Ctrl Pts',(216.109032424958,7.62991562244628,9.42630431063069));
#36264=CARTESIAN_POINT('Ctrl Pts',(216.227505576616,2.22128381937299,11.9221107005453));
#36265=CARTESIAN_POINT('Ctrl Pts',(216.345978728275,-3.72325552497568,11.5415854048741));
#36266=CARTESIAN_POINT('Ctrl Pts',(216.464451879933,-8.76952122390942,8.37653406043739));
#36267=CARTESIAN_POINT('Ctrl Pts',(216.582925031591,-11.7000498359031,3.19055781951202));
#36268=CARTESIAN_POINT('Ctrl Pts',(216.70139818325,-11.8078212271973,-2.76517327283705));
#36269=CARTESIAN_POINT('Ctrl Pts',(216.819871334908,-9.06683444247781,-8.05377790573855));
#36270=CARTESIAN_POINT('Ctrl Pts',(216.938344486566,-4.13838070245931,-11.3993258802342));
#36271=CARTESIAN_POINT('Ctrl Pts',(217.056817638225,1.78849989673574,-11.9946693777545));
#36272=CARTESIAN_POINT('Ctrl Pts',(217.175290789883,7.2838865220984,-9.69617566339728));
#36273=CARTESIAN_POINT('Ctrl Pts',(217.293763941541,11.0219606946616,-5.05837995880107));
#36274=CARTESIAN_POINT('Ctrl Pts',(217.4122370932,12.1008736180437,0.799801876966326));
#36275=CARTESIAN_POINT('Ctrl Pts',(217.530710244858,10.2603264655135,6.46502329333376));
#36276=CARTESIAN_POINT('Ctrl Pts',(217.649183396516,5.94437014605935,10.5704914232454));
#36277=CARTESIAN_POINT('Ctrl Pts',(217.767656548175,0.19427346074058,12.1257199037712));
#36278=CARTESIAN_POINT('Ctrl Pts',(217.886129699833,-5.60269369280611,10.755493886701));
#36279=CARTESIAN_POINT('Ctrl Pts',(218.004602851491,-10.0479534349698,6.79039447535502));
#36280=CARTESIAN_POINT('Ctrl Pts',(218.12307600315,-12.0690411855952,1.18704263726627));
#36281=CARTESIAN_POINT('Ctrl Pts',(218.241549154808,-11.1783487616574,-4.70269543187866));
#36282=CARTESIAN_POINT('Ctrl Pts',(218.360022306466,-7.59076486076366,-9.45785991600705));
#36283=CARTESIAN_POINT('Ctrl Pts',(218.478495458124,-2.17183095521254,-11.9312185322559));
#36284=CARTESIAN_POINT('Ctrl Pts',(218.596968609783,3.77107948007088,-11.5260481049111));
#36285=CARTESIAN_POINT('Ctrl Pts',(218.715441761441,8.80417824950912,-8.34010016212016));
#36286=CARTESIAN_POINT('Ctrl Pts',(218.833914913099,11.7131785684463,-3.14201737492898));
#36287=CARTESIAN_POINT('Ctrl Pts',(218.952388064758,11.7962542252798,2.8141093823934));
#36288=CARTESIAN_POINT('Ctrl Pts',(219.070861216416,9.03336236373215,8.0913033418722));
#36289=CARTESIAN_POINT('Ctrl Pts',(219.189334368074,4.09107903060885,11.4163872443638));
#36290=CARTESIAN_POINT('Ctrl Pts',(219.307807519733,-1.8382191492073,11.987150443861));
#36291=CARTESIAN_POINT('Ctrl Pts',(219.426280671391,-7.32402807100668,9.66589044452053));
#36292=CARTESIAN_POINT('Ctrl Pts',(219.544753823049,-11.0428399867738,5.01263508976042));
#36293=CARTESIAN_POINT('Ctrl Pts',(219.663226974708,-12.0974532932881,-0.849970007145037));
#36294=CARTESIAN_POINT('Ctrl Pts',(219.781700126366,-10.2334317465363,-6.50751104396671));
#36295=CARTESIAN_POINT('Ctrl Pts',(219.900173278024,-5.90048958874147,-10.5950483214781));
#36296=CARTESIAN_POINT('Ctrl Pts',(220.018646429683,-0.143993849436442,
-12.1264210667714));
#36297=CARTESIAN_POINT('Ctrl Pts',(220.137119581341,5.64724219684359,-10.7321707342743));
#36298=CARTESIAN_POINT('Ctrl Pts',(220.255592732999,10.0760223966742,-6.74867274049521));
#36299=CARTESIAN_POINT('Ctrl Pts',(220.374065884658,12.0738600392668,-1.13699065996796));
#36300=CARTESIAN_POINT('Ctrl Pts',(220.492539036316,11.1587520687127,4.74900741041341));
#36301=CARTESIAN_POINT('Ctrl Pts',(220.611012187974,7.55148645936778,9.48924755630021));
#36302=CARTESIAN_POINT('Ctrl Pts',(220.729485339633,2.12233476463566,11.9401324320201));
#36303=CARTESIAN_POINT('Ctrl Pts',(220.847958491291,-3.81882609063897,11.5102892545281));
#36304=CARTESIAN_POINT('Ctrl Pts',(220.966431642949,-8.83871002437373,8.30357180650651));
#36305=CARTESIAN_POINT('Ctrl Pts',(221.084904794608,-11.7260511632741,3.09332134717786));
#36306=CARTESIAN_POINT('Ctrl Pts',(221.203377946266,-11.7845969010132,-2.86277702704783));
#36307=CARTESIAN_POINT('Ctrl Pts',(221.321851097924,-8.99947916585132,-8.12909058266712));
#36308=CARTESIAN_POINT('Ctrl Pts',(221.40083319903,-5.69586276335608,-10.330631930925));
#36309=CARTESIAN_POINT('Ctrl Pts',(221.440324249582,-3.88078001816469,-10.9725894971567));
#36310=CARTESIAN_POINT('Ctrl Pts',(203.834675750418,6.59052307073188,-9.24336091171122));
#36311=CARTESIAN_POINT('Ctrl Pts',(203.87416680097,8.11955729759066,-8.15315839291918));
#36312=CARTESIAN_POINT('Ctrl Pts',(203.953148902076,10.6245887795654,-5.20027974474125));
#36313=CARTESIAN_POINT('Ctrl Pts',(204.071622053734,11.8189513632536,0.486505596500501));
#36314=CARTESIAN_POINT('Ctrl Pts',(204.190095205392,10.1616331768082,6.05494567902541));
#36315=CARTESIAN_POINT('Ctrl Pts',(204.308568357051,6.05281639955519,10.1630507991643));
#36316=CARTESIAN_POINT('Ctrl Pts',(204.427041508709,0.483646122609916,11.8189872186854));
#36317=CARTESIAN_POINT('Ctrl Pts',(204.545514660367,-5.20218526685233,10.6235810459546));
#36318=CARTESIAN_POINT('Ctrl Pts',(204.663987812026,-9.63294727221344,6.86507442242633));
#36319=CARTESIAN_POINT('Ctrl Pts',(204.782460963684,-11.7396564004687,1.45032314392112));
#36320=CARTESIAN_POINT('Ctrl Pts',(204.900934115342,-11.0140553954953,-4.31434549514265));
#36321=CARTESIAN_POINT('Ctrl Pts',(205.019407267001,-7.63119914199956,-9.03812821601569));
#36322=CARTESIAN_POINT('Ctrl Pts',(205.137880418659,-2.40723828876296,-11.5813724035012));
#36323=CARTESIAN_POINT('Ctrl Pts',(205.256353570317,3.39749381456364,-11.3304902038307));
#36324=CARTESIAN_POINT('Ctrl Pts',(205.374826721976,8.3825454964294,-8.34601147129938));
#36325=CARTESIAN_POINT('Ctrl Pts',(205.493299873634,11.3452220258881,-3.34797142891857));
#36326=CARTESIAN_POINT('Ctrl Pts',(205.611773025292,11.5707471580529,2.4578009709673));
#36327=CARTESIAN_POINT('Ctrl Pts',(205.730246176951,9.00471068375088,7.67060370603969));
#36328=CARTESIAN_POINT('Ctrl Pts',(205.848719328609,4.26619524205395,11.0327944617666));
#36329=CARTESIAN_POINT('Ctrl Pts',(205.967192480267,-1.50158362617033,11.733210226529));
#36330=CARTESIAN_POINT('Ctrl Pts',(206.085665631925,-6.9070900200322,9.60286847811134));
#36331=CARTESIAN_POINT('Ctrl Pts',(206.204138783584,-10.6461899873718,5.15573606010141));
#36332=CARTESIAN_POINT('Ctrl Pts',(206.322611935242,-11.8167872494313,-0.535270650419746));
#36333=CARTESIAN_POINT('Ctrl Pts',(206.441085086901,-10.1364631903243,-6.09713781671562));
#36334=CARTESIAN_POINT('Ctrl Pts',(206.559558238559,-6.01061325199916,-10.1880078475748));
#36335=CARTESIAN_POINT('Ctrl Pts',(206.678031390217,-0.43464111792699,-11.8209163208462));
#36336=CARTESIAN_POINT('Ctrl Pts',(206.796504541875,5.24619265101169,-10.6019072923227));
#36337=CARTESIAN_POINT('Ctrl Pts',(206.914977693534,9.66132854734208,-6.82507921321143));
#36338=CARTESIAN_POINT('Ctrl Pts',(207.033450845192,11.7455696781712,-1.40163065804246));
#36339=CARTESIAN_POINT('Ctrl Pts',(207.15192399685,10.9960714587182,4.35997569272144));
#36340=CARTESIAN_POINT('Ctrl Pts',(207.270397148509,7.59365803422165,9.06969311639776));
#36341=CARTESIAN_POINT('Ctrl Pts',(207.388870300167,2.3591965972595,11.5912539003263));
#36342=CARTESIAN_POINT('Ctrl Pts',(207.507343451825,-3.44444525545874,11.3163056007024));
#36343=CARTESIAN_POINT('Ctrl Pts',(207.625816603484,-8.41707930457644,8.31118231943059));
#36344=CARTESIAN_POINT('Ctrl Pts',(207.744289755142,-11.3590065005247,3.30090092056398));
#36345=CARTESIAN_POINT('Ctrl Pts',(207.8627629068,-11.5604566840645,-2.50575673643968));
#36346=CARTESIAN_POINT('Ctrl Pts',(207.981236058459,-8.97282792886425,-7.70787483845822));
#36347=CARTESIAN_POINT('Ctrl Pts',(208.099709210117,-4.22041225552873,-11.0503889506083));
#36348=CARTESIAN_POINT('Ctrl Pts',(208.218182361775,1.55022123189376,-11.7268832047791));
#36349=CARTESIAN_POINT('Ctrl Pts',(208.336655513433,6.94684792127837,-9.57414641234265));
#36350=CARTESIAN_POINT('Ctrl Pts',(208.455128665092,10.6674761828003,-5.11154844012378));
#36351=CARTESIAN_POINT('Ctrl Pts',(208.57360181675,11.8144662253433,0.584263105599529));
#36352=CARTESIAN_POINT('Ctrl Pts',(208.692074968409,10.111094917804,6.13911517480345));
#36353=CARTESIAN_POINT('Ctrl Pts',(208.810548120067,5.96831808732183,10.2128426392895));
#36354=CARTESIAN_POINT('Ctrl Pts',(208.929021271725,0.385623204121608,11.8226168977425));
#36355=CARTESIAN_POINT('Ctrl Pts',(209.047494423383,-5.29010723868483,10.5800633726627));
#36356=CARTESIAN_POINT('Ctrl Pts',(209.165967575042,-9.68954496345093,6.78496086706518));
#36357=CARTESIAN_POINT('Ctrl Pts',(209.2844407267,-11.7512804224591,1.3529168485436));
#36358=CARTESIAN_POINT('Ctrl Pts',(209.402913878358,-10.9778987554555,-4.40553225857115));
#36359=CARTESIAN_POINT('Ctrl Pts',(209.521387030017,-7.55598623476468,-9.10110144907693));
#36360=CARTESIAN_POINT('Ctrl Pts',(209.639860181675,-2.31111441023934,-11.6009364169073));
#36361=CARTESIAN_POINT('Ctrl Pts',(209.758333333333,3.49133750846188,-11.3019262945903));
#36362=CARTESIAN_POINT('Ctrl Pts',(209.876806484992,8.45146838578882,-8.27621034594672));
#36363=CARTESIAN_POINT('Ctrl Pts',(209.99527963665,11.3725956908155,-3.25377362758823));
#36364=CARTESIAN_POINT('Ctrl Pts',(210.113752788308,11.5499674516705,2.55366940532554));
#36365=CARTESIAN_POINT('Ctrl Pts',(210.232225939967,8.94079090885937,7.74501345966559));
#36366=CARTESIAN_POINT('Ctrl Pts',(210.350699091625,4.17455670811409,11.0677934502358));
#36367=CARTESIAN_POINT('Ctrl Pts',(210.469172243283,-1.59883218481789,11.7203545684904));
#36368=CARTESIAN_POINT('Ctrl Pts',(210.587645394941,-6.98648638792551,9.54525974071292));
#36369=CARTESIAN_POINT('Ctrl Pts',(210.7061185466,-10.6885789758751,5.06727293944427));
#36370=CARTESIAN_POINT('Ctrl Pts',(210.824591698258,-11.8119420792218,-0.633245515935656));
#36371=CARTESIAN_POINT('Ctrl Pts',(210.943064849916,-10.0855528086691,-6.18098698509304));
#36372=CARTESIAN_POINT('Ctrl Pts',(211.061538001575,-5.92592031140351,-10.2375018451397));
#36373=CARTESIAN_POINT('Ctrl Pts',(211.180011153233,-0.336598660423963,
-11.8241142124112));
#36374=CARTESIAN_POINT('Ctrl Pts',(211.298484304891,5.33393087535229,-10.5580375536038));
#36375=CARTESIAN_POINT('Ctrl Pts',(211.41695745655,9.71759479053014,-6.74472586940382));
#36376=CARTESIAN_POINT('Ctrl Pts',(211.535430608208,11.7567891310036,-1.30417977881064));
#36377=CARTESIAN_POINT('Ctrl Pts',(211.653903759866,10.9595373129366,4.45101308161348));
#36378=CARTESIAN_POINT('Ctrl Pts',(211.772376911525,7.518184527822,9.13235330963281));
#36379=CARTESIAN_POINT('Ctrl Pts',(211.890850063183,2.26299248902007,11.6104194825588));
#36380=CARTESIAN_POINT('Ctrl Pts',(212.009323214841,-3.53816973609404,11.2873526783268));
#36381=CARTESIAN_POINT('Ctrl Pts',(212.1277963665,-8.48571216379742,8.24109608241064));
#36382=CARTESIAN_POINT('Ctrl Pts',(212.246269518158,-11.3859893559603,3.20659039359594));
#36383=CARTESIAN_POINT('Ctrl Pts',(212.364742669816,-11.5392796446386,-2.60153816984724));
#36384=CARTESIAN_POINT('Ctrl Pts',(212.483215821474,-8.90860017289598,-7.78201892350702));
#36385=CARTESIAN_POINT('Ctrl Pts',(212.601688973133,-4.1286293889745,-11.0850076650781));
#36386=CARTESIAN_POINT('Ctrl Pts',(212.720162124791,1.64741564956743,-11.7136244281565));
#36387=CARTESIAN_POINT('Ctrl Pts',(212.838635276449,7.02600473830304,-9.51620896069891));
#36388=CARTESIAN_POINT('Ctrl Pts',(212.957108428108,10.7094980038693,-5.02291031887514));
#36389=CARTESIAN_POINT('Ctrl Pts',(213.075581579766,11.8092148544223,0.682217039098379));
#36390=CARTESIAN_POINT('Ctrl Pts',(213.194054731424,10.0598373020762,6.22275252778859));
#36391=CARTESIAN_POINT('Ctrl Pts',(213.312527883083,5.88342065316515,10.261985041124));
#36392=CARTESIAN_POINT('Ctrl Pts',(213.431001034741,0.287568329700688,11.8254082391305));
#36393=CARTESIAN_POINT('Ctrl Pts',(213.549474186399,-5.3776628075716,10.5358302138182));
#36394=CARTESIAN_POINT('Ctrl Pts',(213.667947338058,-9.74547754632755,6.70437491197867));
#36395=CARTESIAN_POINT('Ctrl Pts',(213.786420489716,-11.7620957090959,1.25542028676107));
#36396=CARTESIAN_POINT('Ctrl Pts',(213.904893641374,-10.9409874468431,-4.49641737991101));
#36397=CARTESIAN_POINT('Ctrl Pts',(214.023366793033,-7.48025356330558,-9.16344816076338));
#36398=CARTESIAN_POINT('Ctrl Pts',(214.141839944691,-2.21483166094538,-11.6197029342414));
#36399=CARTESIAN_POINT('Ctrl Pts',(214.260313096349,3.58494113318469,-11.2725850024714));
#36400=CARTESIAN_POINT('Ctrl Pts',(214.378786248008,8.51981004986064,-8.20584013252983));
#36401=CARTESIAN_POINT('Ctrl Pts',(214.497259399666,11.3991872656865,-3.15935202979238));
#36402=CARTESIAN_POINT('Ctrl Pts',(214.615732551324,11.5283934467207,2.64936220701343));
#36403=CARTESIAN_POINT('Ctrl Pts',(214.734205702982,8.87625627441841,7.81889059376015));
#36404=CARTESIAN_POINT('Ctrl Pts',(214.852678854641,4.08263108772274,11.1020312991769));
#36405=CARTESIAN_POINT('Ctrl Pts',(214.971152006299,-1.69597079086341,11.7066928994863));
#36406=CARTESIAN_POINT('Ctrl Pts',(215.089625157957,-7.06540229298547,9.48699457176081));
#36407=CARTESIAN_POINT('Ctrl Pts',(215.208098309616,-10.7302329071292,4.9784613411278));
#36408=CARTESIAN_POINT('Ctrl Pts',(215.326571461274,-11.8062845978329,-0.731176833136949));
#36409=CARTESIAN_POINT('Ctrl Pts',(215.445044612932,-10.0339488401432,-6.26441108482937));
#36410=CARTESIAN_POINT('Ctrl Pts',(215.563517764591,-5.84081984328888,-10.2862918063113));
#36411=CARTESIAN_POINT('Ctrl Pts',(215.681990916249,-0.238533054913557,
-11.8264989556528));
#36412=CARTESIAN_POINT('Ctrl Pts',(215.800464067907,5.42130228347449,-10.5134417351093));
#36413=CARTESIAN_POINT('Ctrl Pts',(215.918937219566,9.77319275146448,-6.66390868853002));
#36414=CARTESIAN_POINT('Ctrl Pts',(216.037410371224,11.7672000655017,-1.20663921070012));
#36415=CARTESIAN_POINT('Ctrl Pts',(216.155883522882,10.9222494760965,4.54174437284327));
#36416=CARTESIAN_POINT('Ctrl Pts',(216.274356674541,7.44219399334947,9.19438546786551));
#36417=CARTESIAN_POINT('Ctrl Pts',(216.392829826199,2.16663275402798,11.6287866123477));
#36418=CARTESIAN_POINT('Ctrl Pts',(216.511302977857,-3.63165089560916,11.2576235209197));
#36419=CARTESIAN_POINT('Ctrl Pts',(216.629776129516,-8.55376145774527,8.17044310244772));
#36420=CARTESIAN_POINT('Ctrl Pts',(216.748249281174,-11.412189193087,3.11205934833045));
#36421=CARTESIAN_POINT('Ctrl Pts',(216.866722432833,-11.5173090450793,-2.69714069460188));
#36422=CARTESIAN_POINT('Ctrl Pts',(216.98519558449,-8.84375976950426,-7.85562783650302));
#36423=CARTESIAN_POINT('Ctrl Pts',(217.103668736149,-4.03656259519177,-11.1188640598508));
#36424=CARTESIAN_POINT('Ctrl Pts',(217.222141887807,1.74449677391393,-11.6995601016511));
#36425=CARTESIAN_POINT('Ctrl Pts',(217.340615039466,7.10467837462401,-9.45761707617162));
#36426=CARTESIAN_POINT('Ctrl Pts',(217.459088191124,10.7507833291668,-4.93392677039839));
#36427=CARTESIAN_POINT('Ctrl Pts',(217.577561342782,11.8031513598328,0.780124056302488));
#36428=CARTESIAN_POINT('Ctrl Pts',(217.69603449444,10.0078878679614,6.30596193999415));
#36429=CARTESIAN_POINT('Ctrl Pts',(217.814507646099,5.79811861419576,10.3104217228036));
#36430=CARTESIAN_POINT('Ctrl Pts',(217.932980797757,0.189493679109268,11.8273863432255));
#36431=CARTESIAN_POINT('Ctrl Pts',(218.051453949416,-5.46484855278258,10.4908725023946));
#36432=CARTESIAN_POINT('Ctrl Pts',(218.169927101073,-9.80073992944261,6.62332789477926));
#36433=CARTESIAN_POINT('Ctrl Pts',(218.288400252732,-11.7721021124642,1.15783738930527));
#36434=CARTESIAN_POINT('Ctrl Pts',(218.40687340439,-10.9033237228513,-4.58699328112077));
#36435=CARTESIAN_POINT('Ctrl Pts',(218.525346556049,-7.4040064723011,-9.22516469904043));
#36436=CARTESIAN_POINT('Ctrl Pts',(218.643819707707,-2.11839659692998,-11.6376703607144));
#36437=CARTESIAN_POINT('Ctrl Pts',(218.762292859365,3.67829822029263,-11.2424684908802));
#36438=CARTESIAN_POINT('Ctrl Pts',(218.880766011023,8.58756580375752,-8.13490560077299));
#36439=CARTESIAN_POINT('Ctrl Pts',(218.999239162682,11.4249949145797,-3.06471316221435));
#36440=CARTESIAN_POINT('Ctrl Pts',(219.11771231434,11.5060266303775,2.74487281099996));
#36441=CARTESIAN_POINT('Ctrl Pts',(219.236185465999,8.81111121666141,7.89223002048656));
#36442=CARTESIAN_POINT('Ctrl Pts',(219.354658617657,3.99042470382567,11.135505656944));
#36443=CARTESIAN_POINT('Ctrl Pts',(219.473131769315,-1.79299276527314,11.6922261588623));
#36444=CARTESIAN_POINT('Ctrl Pts',(219.591604920974,-7.14383230619438,9.42807697570855));
#36445=CARTESIAN_POINT('Ctrl Pts',(219.710078072632,-10.7711489203518,4.8893073792482));
#36446=CARTESIAN_POINT('Ctrl Pts',(219.82855122429,-11.799815186589,-0.82905788146501));
#36447=CARTESIAN_POINT('Ctrl Pts',(219.947024375948,-9.98165484967794,-6.34740434882255));
#36448=CARTESIAN_POINT('Ctrl Pts',(220.065497527607,-5.75531766641918,-10.3343744386089));
#36449=CARTESIAN_POINT('Ctrl Pts',(220.183970679265,-0.140451115632587,
-11.8280702552538));
#36450=CARTESIAN_POINT('Ctrl Pts',(220.302443830923,5.50830101353917,-10.4681231780922));
#36451=CARTESIAN_POINT('Ctrl Pts',(220.420916982582,9.82811830012625,-6.58263265515534));
#36452=CARTESIAN_POINT('Ctrl Pts',(220.53939013424,11.7768024061011,-1.10901685927098));
#36453=CARTESIAN_POINT('Ctrl Pts',(220.657863285898,10.8842091745733,4.63216582896095));
#36454=CARTESIAN_POINT('Ctrl Pts',(220.776336437557,7.36569445190642,9.25578009763907));
#36455=CARTESIAN_POINT('Ctrl Pts',(220.894809589215,2.07011817939136,11.6463649485139));
#36456=CARTESIAN_POINT('Ctrl Pts',(221.013282740873,-3.72487010338492,11.2270973613073));
#36457=CARTESIAN_POINT('Ctrl Pts',(221.131755892532,-8.62124798062474,8.09927596576955));
#36458=CARTESIAN_POINT('Ctrl Pts',(221.25022904419,-11.4375508002076,3.01721522080027));
#36459=CARTESIAN_POINT('Ctrl Pts',(221.368702195848,-11.4946561155609,-2.79234306763717));
#36460=CARTESIAN_POINT('Ctrl Pts',(221.487175347506,-8.77806165959916,-7.92908756785469));
#36461=CARTESIAN_POINT('Ctrl Pts',(221.566157448612,-5.5557253503153,-10.0764635820684));
#36462=CARTESIAN_POINT('Ctrl Pts',(221.605648499165,-3.78529975557396,-10.7026268294495));
#36463=CARTESIAN_POINT('Ctrl Pts',(204.,6.42428395783811,-9.01020671414169));
#36464=CARTESIAN_POINT('Ctrl Pts',(204.039491050553,7.91474988128163,-7.9475034238105));
#36465=CARTESIAN_POINT('Ctrl Pts',(204.118473151658,10.3565945407743,-5.06910807865537));
#36466=CARTESIAN_POINT('Ctrl Pts',(204.236946303317,11.5208305663343,0.474233997127887));
#36467=CARTESIAN_POINT('Ctrl Pts',(204.355419454975,9.90531651320884,5.90221595067179));
#36468=CARTESIAN_POINT('Ctrl Pts',(204.473892606633,5.90014038006902,9.90669837751048));
#36469=CARTESIAN_POINT('Ctrl Pts',(204.592365758292,0.471446650502101,11.5208655173499));
#36470=CARTESIAN_POINT('Ctrl Pts',(204.71083890995,-5.07096553594642,10.3556122261992));
#36471=CARTESIAN_POINT('Ctrl Pts',(204.829312061608,-9.38996616253539,6.69191003627886));
#36472=CARTESIAN_POINT('Ctrl Pts',(204.947785213267,-11.4435357367905,1.41374024598308));
#36473=CARTESIAN_POINT('Ctrl Pts',(205.066258364925,-10.7362372650283,-4.20552060216643));
#36474=CARTESIAN_POINT('Ctrl Pts',(205.184731516583,-7.43871005394589,-8.8101508004562));
#36475=CARTESIAN_POINT('Ctrl Pts',(205.303204668241,-2.34651819820973,-11.2892442895734));
#36476=CARTESIAN_POINT('Ctrl Pts',(205.4216778199,3.31179555484533,-11.0446903333316));
#36477=CARTESIAN_POINT('Ctrl Pts',(205.540150971558,8.17110447541142,-8.13549198319505));
#36478=CARTESIAN_POINT('Ctrl Pts',(205.658624123217,11.0590505604482,-3.26352232004452));
#36479=CARTESIAN_POINT('Ctrl Pts',(205.777097274875,11.2788870549277,2.39580548916746));
#36480=CARTESIAN_POINT('Ctrl Pts',(205.895570426533,8.777576190803,7.47712067870388));
#36481=CARTESIAN_POINT('Ctrl Pts',(206.014043578191,4.15858488930056,10.7545036577774));
#36482=CARTESIAN_POINT('Ctrl Pts',(206.13251672985,-1.46370773570288,11.4372521609064));
#36483=CARTESIAN_POINT('Ctrl Pts',(206.250989881508,-6.73286583398743,9.36064607483558));
#36484=CARTESIAN_POINT('Ctrl Pts',(206.369463033166,-10.377650880505,5.02568796228774));
#36485=CARTESIAN_POINT('Ctrl Pts',(206.487936184825,-11.5187210400399,-0.521769003110613));
#36486=CARTESIAN_POINT('Ctrl Pts',(206.606409336483,-9.8807814135434,-5.94334383542404));
#36487=CARTESIAN_POINT('Ctrl Pts',(206.724882488141,-5.85900176316342,-9.93102591024465));
#36488=CARTESIAN_POINT('Ctrl Pts',(206.8433556398,-0.423677746264986,-11.5227459599084));
#36489=CARTESIAN_POINT('Ctrl Pts',(206.961828791458,5.11386287945728,-10.3344851705362));
#36490=CARTESIAN_POINT('Ctrl Pts',(207.080301943116,9.41763154941819,-6.65292366475841));
#36491=CARTESIAN_POINT('Ctrl Pts',(207.198775094774,11.4492998581925,-1.36627597758734));
#36492=CARTESIAN_POINT('Ctrl Pts',(207.317248246433,10.7187069544147,4.24999982531037));
#36493=CARTESIAN_POINT('Ctrl Pts',(207.435721398091,7.40211588169753,8.8409195089455));
#36494=CARTESIAN_POINT('Ctrl Pts',(207.554194549749,2.29968830857567,11.298876535884));
#36495=CARTESIAN_POINT('Ctrl Pts',(207.672667701408,-3.35756269431251,11.0308635221138));
#36496=CARTESIAN_POINT('Ctrl Pts',(207.791140853066,-8.20476720404479,8.10154136057916));
#36497=CARTESIAN_POINT('Ctrl Pts',(207.909614004724,-11.0724873360008,3.2176391164711));
#36498=CARTESIAN_POINT('Ctrl Pts',(208.028087156383,-11.2688561474788,-2.4425516201655));
#36499=CARTESIAN_POINT('Ctrl Pts',(208.146560308041,-8.74649764535955,-7.51345168544144));
#36500=CARTESIAN_POINT('Ctrl Pts',(208.265033459699,-4.11395673115298,-10.771654343876));
#36501=CARTESIAN_POINT('Ctrl Pts',(208.383506611358,1.51111850823841,-11.4310847317218));
#36502=CARTESIAN_POINT('Ctrl Pts',(208.501979763016,6.77162088338667,-9.33264849340337));
#36503=CARTESIAN_POINT('Ctrl Pts',(208.620452914674,10.3984001537186,-4.9826149292203));
#36504=CARTESIAN_POINT('Ctrl Pts',(208.738926066332,11.5164585613786,0.569525674392788));
#36505=CARTESIAN_POINT('Ctrl Pts',(208.857399217991,9.85605302940134,5.98426235816675));
#36506=CARTESIAN_POINT('Ctrl Pts',(208.975872369649,5.817773450173,9.95523427008149));
#36507=CARTESIAN_POINT('Ctrl Pts',(209.094345521308,0.375896258524645,11.5244036415153));
#36508=CARTESIAN_POINT('Ctrl Pts',(209.212818672966,-5.15666976717709,10.3131922411068));
#36509=CARTESIAN_POINT('Ctrl Pts',(209.331291824624,-9.44513623567911,6.61381726230806));
#36510=CARTESIAN_POINT('Ctrl Pts',(209.449764976282,-11.4548665548753,1.31879092343762));
#36511=CARTESIAN_POINT('Ctrl Pts',(209.568238127941,-10.7009926387546,-4.29440727400929));
#36512=CARTESIAN_POINT('Ctrl Pts',(209.686711279599,-7.36539431433226,-8.87153559898989));
#36513=CARTESIAN_POINT('Ctrl Pts',(209.805184431257,-2.25281894488235,-11.3083148210209));
#36514=CARTESIAN_POINT('Ctrl Pts',(209.923657582916,3.40327213884093,-11.0168469190931));
#36515=CARTESIAN_POINT('Ctrl Pts',(210.042130734574,8.23828885633043,-8.06745151887539));
#36516=CARTESIAN_POINT('Ctrl Pts',(210.160603886232,11.0857337530526,-3.17170056060973));
#36517=CARTESIAN_POINT('Ctrl Pts',(210.279077037891,11.2586314950991,2.48925574164375));
#36518=CARTESIAN_POINT('Ctrl Pts',(210.397550189549,8.71526872597554,7.54965352342579));
#36519=CARTESIAN_POINT('Ctrl Pts',(210.516023341207,4.0692578423892,10.7886198330415));
#36520=CARTESIAN_POINT('Ctrl Pts',(210.634496492866,-1.55850330026388,11.4247207735161));
#36521=CARTESIAN_POINT('Ctrl Pts',(210.752969644524,-6.81025951080084,9.30449045812232));
#36522=CARTESIAN_POINT('Ctrl Pts',(210.871442796182,-10.4189706507126,4.9394562321506));
#36523=CARTESIAN_POINT('Ctrl Pts',(210.989915947841,-11.5139980842265,-0.617272554202086));
#36524=CARTESIAN_POINT('Ctrl Pts',(211.108389099499,-9.83115519349314,-6.02507799544502));
#36525=CARTESIAN_POINT('Ctrl Pts',(211.226862251157,-5.77644511420377,-9.97927147302517));
#36526=CARTESIAN_POINT('Ctrl Pts',(211.345335402816,-0.328108308124205,
-11.5258631879735));
#36527=CARTESIAN_POINT('Ctrl Pts',(211.463808554474,5.19938799803607,-10.2917220005022));
#36528=CARTESIAN_POINT('Ctrl Pts',(211.582281706132,9.47247853494596,-6.57459715075616));
#36529=CARTESIAN_POINT('Ctrl Pts',(211.700754857791,11.460236311957,-1.27128319576909));
#36530=CARTESIAN_POINT('Ctrl Pts',(211.819228009449,10.6830943445901,4.33874089043461));
#36531=CARTESIAN_POINT('Ctrl Pts',(211.937701161107,7.32854611626294,8.90199916375812));
#36532=CARTESIAN_POINT('Ctrl Pts',(212.056174312765,2.2059108492439,11.3175586861713));
#36533=CARTESIAN_POINT('Ctrl Pts',(212.174647464424,-3.44892307207615,11.0026409071933));
#36534=CARTESIAN_POINT('Ctrl Pts',(212.293120616082,-8.27166887053497,8.03322297623846));
#36535=CARTESIAN_POINT('Ctrl Pts',(212.411593767741,-11.0987895768778,3.12570747478597));
#36536=CARTESIAN_POINT('Ctrl Pts',(212.530066919398,-11.2482132769208,-2.53591706619991));
#36537=CARTESIAN_POINT('Ctrl Pts',(212.648540071057,-8.68388996795875,-7.58572556280073));
#36538=CARTESIAN_POINT('Ctrl Pts',(212.767013222715,-4.02448899226784,-10.8053998371582));
#36539=CARTESIAN_POINT('Ctrl Pts',(212.885486374374,1.60586129747547,-11.4181603939958));
#36540=CARTESIAN_POINT('Ctrl Pts',(213.003959526032,6.84878105175381,-9.27617245392087));
#36541=CARTESIAN_POINT('Ctrl Pts',(213.12243267769,10.4393620179098,-4.89621261270018));
#36542=CARTESIAN_POINT('Ctrl Pts',(213.240905829349,11.5113396508456,0.665008821455645));
#36543=CARTESIAN_POINT('Ctrl Pts',(213.359378981007,9.806088333898,6.06579004561915));
#36544=CARTESIAN_POINT('Ctrl Pts',(213.477852132665,5.73501746579043,10.0031371057694));
#36545=CARTESIAN_POINT('Ctrl Pts',(213.596325284323,0.280314716669852,11.5271245742102));
#36546=CARTESIAN_POINT('Ctrl Pts',(213.714798435982,-5.24201683759653,10.2700748178432));
#36547=CARTESIAN_POINT('Ctrl Pts',(213.83327158764,-9.49965797713093,6.5352640044053));
#36548=CARTESIAN_POINT('Ctrl Pts',(213.951744739299,-11.4654090371176,1.22375361136365));
#36549=CARTESIAN_POINT('Ctrl Pts',(214.070217890957,-10.6650123796405,-4.38299991237251));
#36550=CARTESIAN_POINT('Ctrl Pts',(214.188691042615,-7.2915719210082,-8.93230967950104));
#36551=CARTESIAN_POINT('Ctrl Pts',(214.307164194274,-2.15896482813512,-11.3266079724081));
#36552=CARTESIAN_POINT('Ctrl Pts',(214.425637345932,3.4945147091572,-10.9882457306536));
#36553=CARTESIAN_POINT('Ctrl Pts',(214.54411049759,8.30490667276723,-7.99885632114799));
#36554=CARTESIAN_POINT('Ctrl Pts',(214.662583649248,11.1116545830117,-3.0796606497433));
#36555=CARTESIAN_POINT('Ctrl Pts',(214.781056800907,11.2376016720611,2.58253479160174));
#36556=CARTESIAN_POINT('Ctrl Pts',(214.899529952565,8.65236191079344,7.62166718339193));
#36557=CARTESIAN_POINT('Ctrl Pts',(215.018003104223,3.9796509504845,10.8219940677331));
#36558=CARTESIAN_POINT('Ctrl Pts',(215.136476255882,-1.65319168566326,11.4114037059512));
#36559=CARTESIAN_POINT('Ctrl Pts',(215.25494940754,-6.88718484395786,9.24769496766087));
#36560=CARTESIAN_POINT('Ctrl Pts',(215.373422559198,-10.4595739047283,4.85288481434185));
#36561=CARTESIAN_POINT('Ctrl Pts',(215.491895710856,-11.5084833069413,-0.712733655440043));
#36562=CARTESIAN_POINT('Ctrl Pts',(215.610368862515,-9.7808528815819,-6.10639780874076));
#36563=CARTESIAN_POINT('Ctrl Pts',(215.728842014173,-5.6934912171844,-10.0268307580006));
#36564=CARTESIAN_POINT('Ctrl Pts',(215.847315165831,-0.232516305860531,
-11.5281877785388));
#36565=CARTESIAN_POINT('Ctrl Pts',(215.96578831749,5.28455555295532,-10.2482510653024));
#36566=CARTESIAN_POINT('Ctrl Pts',(216.084261469148,9.52667409494713,-6.4958184994969));
#36567=CARTESIAN_POINT('Ctrl Pts',(216.202734620806,11.4703846414241,-1.17620298738114));
#36568=CARTESIAN_POINT('Ctrl Pts',(216.321207772465,10.6467470547827,4.42718357889284));
#36569=CARTESIAN_POINT('Ctrl Pts',(216.439680924123,7.25447236425265,8.96246662510033));
#36570=CARTESIAN_POINT('Ctrl Pts',(216.558154075782,2.11198168868298,11.3354625241501));
#36571=CARTESIAN_POINT('Ctrl Pts',(216.67662722744,-3.54004626624265,10.9736616369653));
#36572=CARTESIAN_POINT('Ctrl Pts',(216.795100379098,-8.33800169158112,7.96435214445806));
#36573=CARTESIAN_POINT('Ctrl Pts',(216.913573530756,-11.124328550271,3.03356087714887));
#36574=CARTESIAN_POINT('Ctrl Pts',(217.032046682415,-11.2267968629613,-2.62910811636671));
#36575=CARTESIAN_POINT('Ctrl Pts',(217.150519834073,-8.62068509653071,-7.65747776726749));
#36576=CARTESIAN_POINT('Ctrl Pts',(217.268992985731,-3.93474448792423,-10.8384022394674));
#36577=CARTESIAN_POINT('Ctrl Pts',(217.38746613739,1.70049365109212,-11.4044508255478));
#36578=CARTESIAN_POINT('Ctrl Pts',(217.505939289048,6.92547022714963,-9.21905848894597));
#36579=CARTESIAN_POINT('Ctrl Pts',(217.624412440706,10.4796059636719,-4.80947358199571));
#36580=CARTESIAN_POINT('Ctrl Pts',(217.742885592365,11.5054291016218,0.760446235638654));
#36581=CARTESIAN_POINT('Ctrl Pts',(217.861358744023,9.75544927040927,6.14690058665455));
#36582=CARTESIAN_POINT('Ctrl Pts',(217.979831895681,5.65186708233216,10.0503520223619));
#36583=CARTESIAN_POINT('Ctrl Pts',(218.098305047339,0.184713897477963,11.5290527826799));
#36584=CARTESIAN_POINT('Ctrl Pts',(218.216778198998,-5.32700341275905,10.2262511180883));
#36585=CARTESIAN_POINT('Ctrl Pts',(218.335251350656,-9.55352642391547,6.4562613142035));
#36586=CARTESIAN_POINT('Ctrl Pts',(218.453724502315,-11.4751630393333,1.12863214134426));
#36587=CARTESIAN_POINT('Ctrl Pts',(218.572197653973,-10.6282986840452,-4.47129113036288));
#36588=CARTESIAN_POINT('Ctrl Pts',(218.690670805631,-7.21724808383853,-8.99246948207381));
#36589=CARTESIAN_POINT('Ctrl Pts',(218.809143957289,-2.06496223864743,-11.3441221891729));
#36590=CARTESIAN_POINT('Ctrl Pts',(218.927617108948,3.58551696051438,-10.9588888768492));
#36591=CARTESIAN_POINT('Ctrl Pts',(219.046090260606,8.37095335800593,-7.92971103942582));
#36592=CARTESIAN_POINT('Ctrl Pts',(219.164563412264,11.1368112607131,-2.98740894949973));
#36593=CARTESIAN_POINT('Ctrl Pts',(219.283036563923,11.2157990354753,2.67563623960653));
#36594=CARTESIAN_POINT('Ctrl Pts',(219.401509715581,8.58886006959068,7.69315669910092));
#36595=CARTESIAN_POINT('Ctrl Pts',(219.519982867239,3.8897703770425,10.8546240695241));
#36596=CARTESIAN_POINT('Ctrl Pts',(219.638456018897,-1.74776638133898,11.3973018738637));
#36597=CARTESIAN_POINT('Ctrl Pts',(219.756929170556,-6.96363654138209,9.19026350689656));
#36598=CARTESIAN_POINT('Ctrl Pts',(219.875402322214,-10.4994578539298,4.76597966873598));
#36599=CARTESIAN_POINT('Ctrl Pts',(219.993875473873,-11.50217707989,-0.808145755784987));
#36600=CARTESIAN_POINT('Ctrl Pts',(220.112348625531,-9.72987795281957,-6.18729765367837));
#36601=CARTESIAN_POINT('Ctrl Pts',(220.230821777189,-5.61014574409689,-10.0737005557397));
#36602=CARTESIAN_POINT('Ctrl Pts',(220.349294928847,-0.136908381828727,
-11.5297194437361));
#36603=CARTESIAN_POINT('Ctrl Pts',(220.467768080506,5.36935983023475,-10.20407562191));
#36604=CARTESIAN_POINT('Ctrl Pts',(220.586241232164,9.58021420357832,-6.41659256981546));
#36605=CARTESIAN_POINT('Ctrl Pts',(220.704714383822,11.4797447729354,-1.08104305857399));
#36606=CARTESIAN_POINT('Ctrl Pts',(220.823187535481,10.6096662804338,4.51532424750848));
#36607=CARTESIAN_POINT('Ctrl Pts',(220.941660687139,7.17990244444507,9.02231263897793));
#36608=CARTESIAN_POINT('Ctrl Pts',(221.060133838797,2.01790159414706,11.3525974650078));
#36609=CARTESIAN_POINT('Ctrl Pts',(221.178606990456,-3.63091411613088,10.9439054680865));
#36610=CARTESIAN_POINT('Ctrl Pts',(221.297080142114,-8.40378593687573,7.89498012503259));
#36611=CARTESIAN_POINT('Ctrl Pts',(221.415553293773,-11.1490504371411,2.94110909442268));
#36612=CARTESIAN_POINT('Ctrl Pts',(221.53402644543,-11.2047153301085,-2.72190910822649));
#36613=CARTESIAN_POINT('Ctrl Pts',(221.652499597089,-8.55664415334701,-7.72908455304227));
#36614=CARTESIAN_POINT('Ctrl Pts',(221.731481698195,-5.41558793727451,-9.82229523321173));
#36615=CARTESIAN_POINT('Ctrl Pts',(221.770972748747,-3.68981949298323,-10.4326641617422));
#36616=CARTESIAN_POINT('Ctrl Pts',(221.275,-3.97626028075622,-11.2425521648637));
#36617=CARTESIAN_POINT('Ctrl Pts',(221.235508949447,-5.83600017639738,-10.5848002797813));
#36618=CARTESIAN_POINT('Ctrl Pts',(221.196017898894,-7.52844842425034,-9.45694693863041));
#36619=CARTESIAN_POINT('Ctrl Pts',(221.156526848342,-8.85027938390384,-7.99370649955156));
#36620=CARTESIAN_POINT('Ctrl Pts',(221.117035797789,-10.1721103435575,-6.53046606047255));
#36621=CARTESIAN_POINT('Ctrl Pts',(221.077544747236,-11.1233240150115,-4.73183852346552));
#36622=CARTESIAN_POINT('Ctrl Pts',(221.038053696683,-11.5889331573844,-2.81541834495975));
#36623=CARTESIAN_POINT('Ctrl Pts',(221.019088080173,-11.8125424135174,-1.8950556382265));
#36624=CARTESIAN_POINT('Ctrl Pts',(221.000122463662,-11.9241513443901,-0.947525116180473));
#36625=CARTESIAN_POINT('Ctrl Pts',(220.981156847152,-11.9240411815327,1.80394148113772E-5));
#36626=CARTESIAN_POINT('Origin',(212.6,0.,0.));
#36627=CARTESIAN_POINT('Origin',(221.275,0.,0.));
#36628=CARTESIAN_POINT('Origin',(158.,0.,0.));
#36629=CARTESIAN_POINT('',(166.,-16.55,-2.02679045258887E-15));
#36630=CARTESIAN_POINT('Origin',(166.,0.,0.));
#36631=CARTESIAN_POINT('',(150.,-16.55,-2.02679045258887E-15));
#36632=CARTESIAN_POINT('',(158.,-16.55,-2.02679045258887E-15));
#36633=CARTESIAN_POINT('Origin',(150.,0.,0.));
#36634=CARTESIAN_POINT('Origin',(150.,22.2,0.));
#36635=CARTESIAN_POINT('',(150.,-22.2,-2.71871589410712E-15));
#36636=CARTESIAN_POINT('Origin',(150.,0.,0.));
#36637=CARTESIAN_POINT('Origin',(150.4,0.,0.));
#36638=CARTESIAN_POINT('',(150.4,-22.6,-2.76770176607302E-15));
#36639=CARTESIAN_POINT('Origin',(221.6,0.,0.));
#36640=CARTESIAN_POINT('',(222.,-11.2,-1.37160441504503E-15));
#36641=CARTESIAN_POINT('Origin',(222.,0.,0.));
#36642=CARTESIAN_POINT('',(221.6,-11.6,-1.42059028701093E-15));
#36643=CARTESIAN_POINT('Origin',(222.,5.05,0.));
#36644=CARTESIAN_POINT('',(222.,-5.05,-6.18446633569413E-16));
#36645=CARTESIAN_POINT('Origin',(222.,0.,0.));
#36646=CARTESIAN_POINT('Origin',(209.,0.,0.));
#36647=CARTESIAN_POINT('',(196.,-5.05,-6.18446633569413E-16));
#36648=CARTESIAN_POINT('',(209.,-5.05,-6.18446633569413E-16));
#36649=CARTESIAN_POINT('Origin',(196.,0.,0.));
#36650=CARTESIAN_POINT('Origin',(196.,17.5,0.));
#36651=CARTESIAN_POINT('',(196.,-17.5,-2.14313189850787E-15));
#36652=CARTESIAN_POINT('Origin',(196.,0.,0.));
#36653=CARTESIAN_POINT('Origin',(181.,0.,0.));
#36654=CARTESIAN_POINT('',(166.,-17.5,-2.14313189850787E-15));
#36655=CARTESIAN_POINT('',(181.,-17.5,-2.14313189850787E-15));
#36656=CARTESIAN_POINT('Origin',(166.,0.,0.));
#36657=CARTESIAN_POINT('Origin',(166.,16.55,0.));
#45203=UNCERTAINTY_MEASURE_WITH_UNIT(LENGTH_MEASURE(0.01),#45237,
'DISTANCE_ACCURACY_VALUE',
'Maximum model space distance between geometric entities at asserted c
onnectivities');
#45214=UNCERTAINTY_MEASURE_WITH_UNIT(LENGTH_MEASURE(0.01),#45237,
'DISTANCE_ACCURACY_VALUE',
'Maximum model space distance between geometric entities at asserted c
onnectivities');
#45225=(
GEOMETRIC_REPRESENTATION_CONTEXT(3)
GLOBAL_UNCERTAINTY_ASSIGNED_CONTEXT((#45203))
GLOBAL_UNIT_ASSIGNED_CONTEXT((#45237,#45239,#45240))
REPRESENTATION_CONTEXT('','3D')
);
#45236=(
GEOMETRIC_REPRESENTATION_CONTEXT(3)
GLOBAL_UNCERTAINTY_ASSIGNED_CONTEXT((#45214))
GLOBAL_UNIT_ASSIGNED_CONTEXT((#45237,#45239,#45240))
REPRESENTATION_CONTEXT('','3D')
);
#45237=(
LENGTH_UNIT()
NAMED_UNIT(*)
SI_UNIT(.MILLI.,.METRE.)
);
#45239=(
NAMED_UNIT(*)
PLANE_ANGLE_UNIT()
SI_UNIT($,.RADIAN.)
);
#45240=(
NAMED_UNIT(*)
SI_UNIT($,.STERADIAN.)
SOLID_ANGLE_UNIT()
);
#45251=SHAPE_DEFINITION_REPRESENTATION(#45272,#45323);
#45272=PRODUCT_DEFINITION_SHAPE('',$,#45345);
#45323=SHAPE_REPRESENTATION('',(#17279),#45225);
#45334=PRODUCT_DEFINITION_CONTEXT('part definition',#45399,'design');
#45345=PRODUCT_DEFINITION('2026-10-25-23-38-26-010',
'16_Fount_Oil_Reservoir',#45366,#45334);
#45366=PRODUCT_DEFINITION_FORMATION('',$,#45411);
#45399=APPLICATION_CONTEXT(
'Core Data for Automotive Mechanical Design Process');
#45400=PRODUCT_CONTEXT('part definition',#45399,'mechanical');
#45411=PRODUCT('2026-10-25-23-38-26-010','16_Fount_Oil_Reservoir',$,(#45400));
#45492=COLOUR_RGB('Off White',0.89,0.88,0.83);
#45493=FILL_AREA_STYLE_COLOUR('',#45492);
#45494=FILL_AREA_STYLE('',(#45493));
#45495=SURFACE_STYLE_FILL_AREA(#45494);
#45496=SURFACE_SIDE_STYLE('',(#45495));
#45497=SURFACE_STYLE_USAGE(.BOTH.,#45496);
#45498=PRESENTATION_STYLE_ASSIGNMENT((#45497));
ENDSEC;
END-ISO-10303-21;
